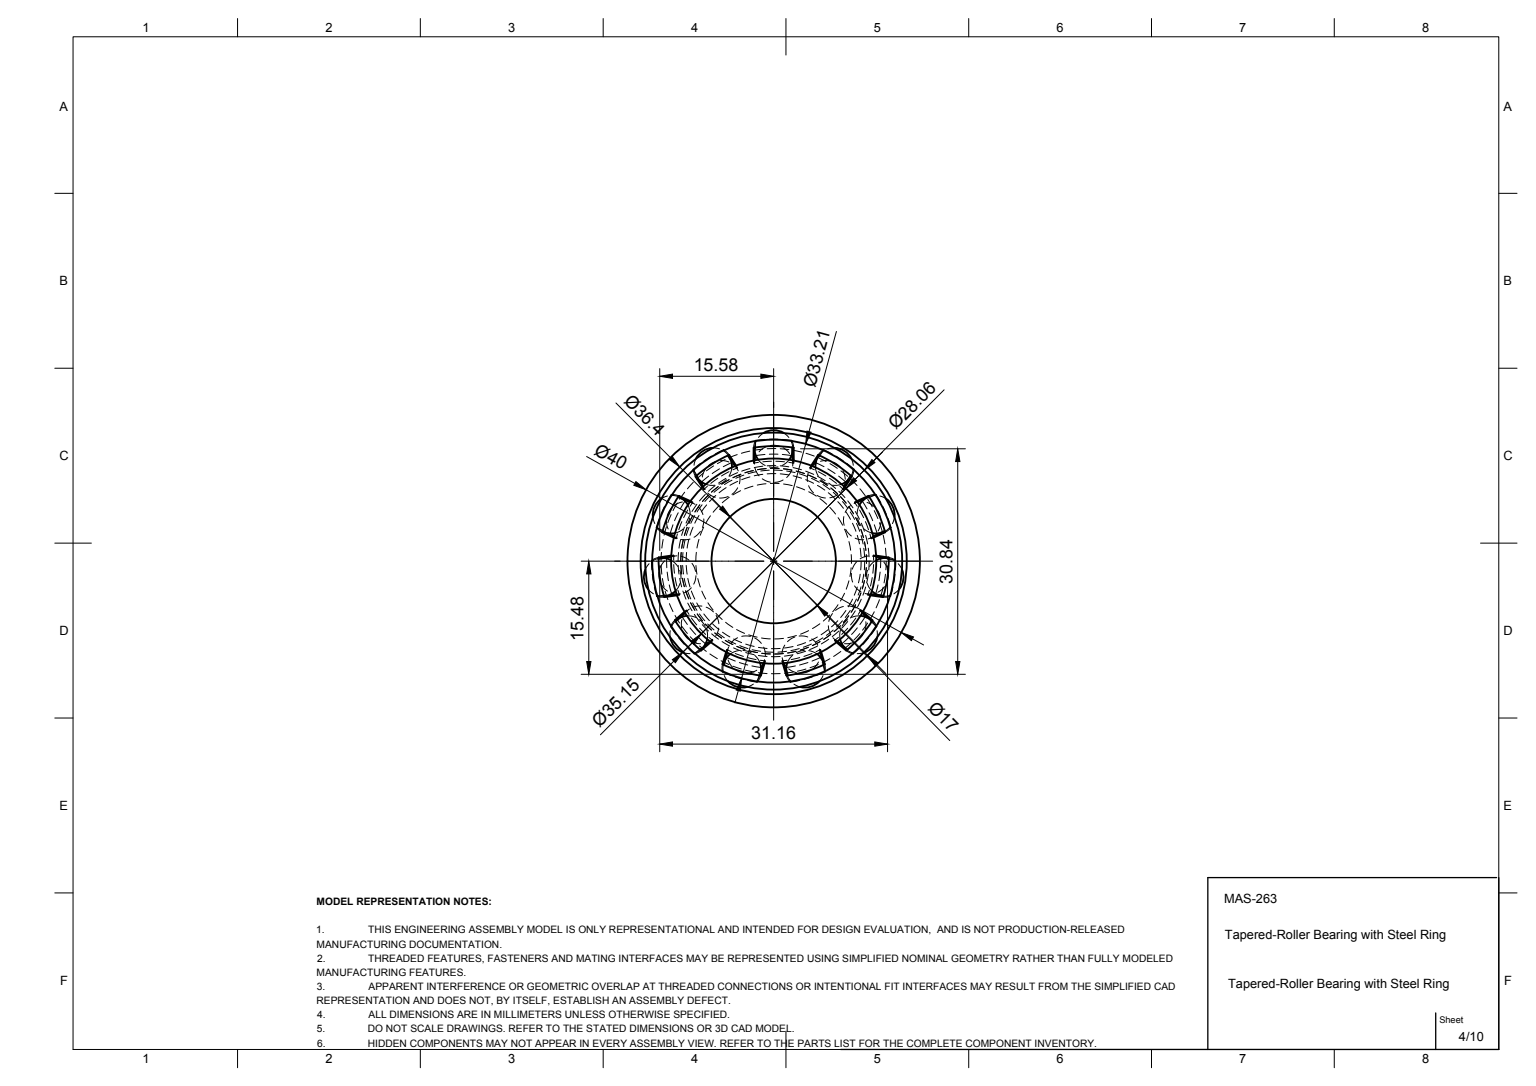
ISO-10303-21;
HEADER;
/* Generated by software containing ST-Developer
 * from STEP Tools, Inc. (www.steptools.com) 
 */

FILE_DESCRIPTION(
/* description */ (''),
/* implementation_level */ '2;1');

FILE_NAME(
/* name */ 'Tapered-Roller Bearing with Steel Ring.step',
/* time_stamp */ '2026-10-12T15:47:30-07:00',
/* author */ (''),
/* organization */ (''),
/* preprocessor_version */ 'ST-DEVELOPER v20.2',
/* originating_system */ 'Autodesk Translation Framework v15.15.0.0',
/* authorisation */ '');

FILE_SCHEMA (('AUTOMOTIVE_DESIGN { 1 0 10303 214 3 1 1 }'));
ENDSEC;

DATA;
#10=MECHANICAL_DESIGN_GEOMETRIC_PRESENTATION_REPRESENTATION('',(#103,#104,#105,#106,#107,#108,#109,#110,#111,#112,#113,#114,#115,#116),#88483);
#72=SHAPE_REPRESENTATION_RELATIONSHIP('SRR','None',#88528,#81);
#81=ADVANCED_BREP_SHAPE_REPRESENTATION('',(#138,#139,#140,#141,#142,#143,
#144,#145,#146,#147,#148,#149,#150,#151),#88482);
#103=STYLED_ITEM('',(#88574),#138);
#104=STYLED_ITEM('',(#88574),#139);
#105=STYLED_ITEM('',(#88574),#140);
#106=STYLED_ITEM('',(#88574),#141);
#107=STYLED_ITEM('',(#88574),#142);
#108=STYLED_ITEM('',(#88574),#143);
#109=STYLED_ITEM('',(#88574),#144);
#110=STYLED_ITEM('',(#88574),#145);
#111=STYLED_ITEM('',(#88574),#146);
#112=STYLED_ITEM('',(#88574),#147);
#113=STYLED_ITEM('',(#88574),#148);
#114=STYLED_ITEM('',(#88574),#149);
#115=STYLED_ITEM('',(#88574),#150);
#116=STYLED_ITEM('',(#88574),#151);
#138=MANIFOLD_SOLID_BREP('Body1',#13013);
#139=MANIFOLD_SOLID_BREP('Body2',#13014);
#140=MANIFOLD_SOLID_BREP('Body3',#13015);
#141=MANIFOLD_SOLID_BREP('Body4',#13016);
#142=MANIFOLD_SOLID_BREP('Body5',#13017);
#143=MANIFOLD_SOLID_BREP('Body6',#13018);
#144=MANIFOLD_SOLID_BREP('Body7',#13019);
#145=MANIFOLD_SOLID_BREP('Body8',#13020);
#146=MANIFOLD_SOLID_BREP('Body9',#13021);
#147=MANIFOLD_SOLID_BREP('Body10',#13022);
#148=MANIFOLD_SOLID_BREP('Body11',#13023);
#149=MANIFOLD_SOLID_BREP('Body12',#13024);
#150=MANIFOLD_SOLID_BREP('Body13',#13025);
#151=MANIFOLD_SOLID_BREP('Body14',#13026);
#185=TOROIDAL_SURFACE('',#14116,19.725,0.275);
#186=TOROIDAL_SURFACE('',#14121,19.725,0.275);
#187=TOROIDAL_SURFACE('',#14141,13.4297712445485,0.500000000000001);
#188=TOROIDAL_SURFACE('',#14288,8.775,0.275);
#189=TOROIDAL_SURFACE('',#14293,8.775,0.275);
#242=ELLIPSE('',#14151,15.0801280312954,14.5834816640173);
#243=ELLIPSE('',#14152,17.3517853554452,16.7803246128912);
#244=ELLIPSE('',#14153,17.3517853554452,16.7803246128912);
#245=ELLIPSE('',#14154,15.0801280312954,14.5834816640173);
#246=ELLIPSE('',#14155,15.0801280312954,14.5834816640173);
#247=ELLIPSE('',#14156,17.3517853554452,16.7803246128912);
#248=ELLIPSE('',#14157,17.3517853554886,16.7803246129121);
#249=ELLIPSE('',#14158,15.0801280313552,14.5834816640461);
#250=ELLIPSE('',#14159,17.351785355493,16.7803246129139);
#251=ELLIPSE('',#14160,15.0801280313139,14.5834816640261);
#252=ELLIPSE('',#14161,17.3517853552649,16.7803246128045);
#253=ELLIPSE('',#14162,15.0801280313118,14.583481664025);
#254=ELLIPSE('',#14163,17.3517853554016,16.7803246128701);
#255=ELLIPSE('',#14164,15.0801280313076,14.583481664023);
#256=ELLIPSE('',#14165,17.3517853554702,16.780324612903);
#257=ELLIPSE('',#14166,15.0801280313709,14.5834816640533);
#258=ELLIPSE('',#14167,17.3517853554861,16.7803246129107);
#259=ELLIPSE('',#14168,15.08012803127,14.583481664005);
#260=ELLIPSE('',#14169,17.3517853554707,16.7803246129033);
#261=ELLIPSE('',#14170,15.0801280312716,14.5834816640059);
#262=ELLIPSE('',#14171,17.3517853553197,16.7803246128311);
#263=ELLIPSE('',#14172,15.0801280311918,14.5834816639677);
#264=ELLIPSE('',#14173,17.3517853552856,16.7803246128146);
#265=ELLIPSE('',#14174,15.0801280313508,14.5834816640437);
#266=ELLIPSE('',#14176,18.421055935048,17.8143800174044);
#267=ELLIPSE('',#14177,16.1493986108983,15.6175370685304);
#268=ELLIPSE('',#14178,16.1493986108983,15.6175370685304);
#269=ELLIPSE('',#14179,18.421055935048,17.8143800174044);
#270=ELLIPSE('',#14180,16.1493986108983,15.6175370685304);
#271=ELLIPSE('',#14181,18.421055935048,17.8143800174044);
#272=ELLIPSE('',#14182,18.4210559352732,17.8143800175124);
#273=ELLIPSE('',#14183,16.1493986107542,15.6175370684613);
#274=ELLIPSE('',#14184,18.4210559346699,17.8143800172222);
#275=ELLIPSE('',#14185,16.1493986106406,15.6175370684066);
#276=ELLIPSE('',#14186,18.421055934899,17.8143800173331);
#277=ELLIPSE('',#14187,16.1493986106858,15.6175370684285);
#278=ELLIPSE('',#14188,18.4210559350675,17.8143800174135);
#279=ELLIPSE('',#14189,16.1493986109801,15.6175370685696);
#280=ELLIPSE('',#14190,18.4210559350065,17.8143800173844);
#281=ELLIPSE('',#14191,16.1493986108565,15.6175370685105);
#282=ELLIPSE('',#14192,18.4210559345343,17.8143800171572);
#283=ELLIPSE('',#14193,16.1493986108155,15.6175370684905);
#284=ELLIPSE('',#14194,18.4210559346994,17.8143800172367);
#285=ELLIPSE('',#14195,16.1493986107405,15.6175370684544);
#286=ELLIPSE('',#14196,18.4210559344304,17.814380017107);
#287=ELLIPSE('',#14197,16.1493986109695,15.6175370685645);
#288=ELLIPSE('',#14198,18.4210559346512,17.8143800172135);
#289=ELLIPSE('',#14199,16.1493986107542,15.6175370684612);
#337=CONICAL_SURFACE('',#14125,15.4,0.249233017184783);
#338=CONICAL_SURFACE('',#14131,12.7058184384753,1.32156330961012);
#339=CONICAL_SURFACE('',#14136,16.6071946160828,1.32156330961011);
#340=CONICAL_SURFACE('',#14146,13.3064408708579,1.32156330961011);
#341=CONICAL_SURFACE('',#14149,12.4591576910941,0.249233017184783);
#342=CONICAL_SURFACE('',#14150,13.0685506725942,0.249233017184784);
#343=CONICAL_SURFACE('',#14175,17.5762965073726,0.249233017184784);
#344=CONICAL_SURFACE('',#14297,10.6410293263727,1.32156330961011);
#345=CONICAL_SURFACE('',#14301,12.6998790237181,0.249233017184785);
#346=CONICAL_SURFACE('',#14304,14.0317131491268,1.32156330961011);
#416=FACE_BOUND('',#2102,.T.);
#417=FACE_BOUND('',#2104,.T.);
#418=FACE_BOUND('',#2111,.T.);
#419=FACE_BOUND('',#2112,.T.);
#420=FACE_BOUND('',#2113,.T.);
#421=FACE_BOUND('',#2114,.T.);
#422=FACE_BOUND('',#2115,.T.);
#423=FACE_BOUND('',#2116,.T.);
#424=FACE_BOUND('',#2117,.T.);
#425=FACE_BOUND('',#2118,.T.);
#426=FACE_BOUND('',#2119,.T.);
#427=FACE_BOUND('',#2120,.T.);
#428=FACE_BOUND('',#2122,.T.);
#429=FACE_BOUND('',#2123,.T.);
#430=FACE_BOUND('',#2124,.T.);
#431=FACE_BOUND('',#2125,.T.);
#432=FACE_BOUND('',#2126,.T.);
#433=FACE_BOUND('',#2127,.T.);
#434=FACE_BOUND('',#2128,.T.);
#435=FACE_BOUND('',#2129,.T.);
#436=FACE_BOUND('',#2130,.T.);
#437=FACE_BOUND('',#2131,.T.);
#438=FACE_BOUND('',#2185,.T.);
#439=FACE_BOUND('',#2187,.T.);
#562=PLANE('',#14129);
#563=PLANE('',#14130);
#564=PLANE('',#14206);
#565=PLANE('',#14207);
#566=PLANE('',#14214);
#567=PLANE('',#14215);
#568=PLANE('',#14222);
#569=PLANE('',#14223);
#570=PLANE('',#14230);
#571=PLANE('',#14231);
#572=PLANE('',#14238);
#573=PLANE('',#14239);
#574=PLANE('',#14246);
#575=PLANE('',#14247);
#576=PLANE('',#14254);
#577=PLANE('',#14255);
#578=PLANE('',#14262);
#579=PLANE('',#14263);
#580=PLANE('',#14270);
#581=PLANE('',#14271);
#582=PLANE('',#14278);
#583=PLANE('',#14279);
#584=PLANE('',#14286);
#585=PLANE('',#14287);
#586=PLANE('',#14311);
#587=PLANE('',#14312);
#588=PLANE('',#14316);
#589=PLANE('',#14317);
#590=PLANE('',#14321);
#591=PLANE('',#14322);
#592=PLANE('',#14326);
#593=PLANE('',#14327);
#594=PLANE('',#14331);
#595=PLANE('',#14332);
#596=PLANE('',#14336);
#597=PLANE('',#14337);
#598=PLANE('',#14341);
#599=PLANE('',#14342);
#600=PLANE('',#14346);
#601=PLANE('',#14347);
#602=PLANE('',#14351);
#603=PLANE('',#14352);
#604=PLANE('',#14356);
#605=PLANE('',#14357);
#606=PLANE('',#14361);
#607=PLANE('',#14362);
#608=PLANE('',#14366);
#609=PLANE('',#14367);
#1362=FACE_OUTER_BOUND('',#2097,.T.);
#1363=FACE_OUTER_BOUND('',#2098,.T.);
#1364=FACE_OUTER_BOUND('',#2099,.T.);
#1365=FACE_OUTER_BOUND('',#2100,.T.);
#1366=FACE_OUTER_BOUND('',#2101,.T.);
#1367=FACE_OUTER_BOUND('',#2103,.T.);
#1368=FACE_OUTER_BOUND('',#2105,.T.);
#1369=FACE_OUTER_BOUND('',#2106,.T.);
#1370=FACE_OUTER_BOUND('',#2107,.T.);
#1371=FACE_OUTER_BOUND('',#2108,.T.);
#1372=FACE_OUTER_BOUND('',#2109,.T.);
#1373=FACE_OUTER_BOUND('',#2110,.T.);
#1374=FACE_OUTER_BOUND('',#2121,.T.);
#1375=FACE_OUTER_BOUND('',#2132,.T.);
#1376=FACE_OUTER_BOUND('',#2133,.T.);
#1377=FACE_OUTER_BOUND('',#2134,.T.);
#1378=FACE_OUTER_BOUND('',#2135,.T.);
#1379=FACE_OUTER_BOUND('',#2136,.T.);
#1380=FACE_OUTER_BOUND('',#2137,.T.);
#1381=FACE_OUTER_BOUND('',#2138,.T.);
#1382=FACE_OUTER_BOUND('',#2139,.T.);
#1383=FACE_OUTER_BOUND('',#2140,.T.);
#1384=FACE_OUTER_BOUND('',#2141,.T.);
#1385=FACE_OUTER_BOUND('',#2142,.T.);
#1386=FACE_OUTER_BOUND('',#2143,.T.);
#1387=FACE_OUTER_BOUND('',#2144,.T.);
#1388=FACE_OUTER_BOUND('',#2145,.T.);
#1389=FACE_OUTER_BOUND('',#2146,.T.);
#1390=FACE_OUTER_BOUND('',#2147,.T.);
#1391=FACE_OUTER_BOUND('',#2148,.T.);
#1392=FACE_OUTER_BOUND('',#2149,.T.);
#1393=FACE_OUTER_BOUND('',#2150,.T.);
#1394=FACE_OUTER_BOUND('',#2151,.T.);
#1395=FACE_OUTER_BOUND('',#2152,.T.);
#1396=FACE_OUTER_BOUND('',#2153,.T.);
#1397=FACE_OUTER_BOUND('',#2154,.T.);
#1398=FACE_OUTER_BOUND('',#2155,.T.);
#1399=FACE_OUTER_BOUND('',#2156,.T.);
#1400=FACE_OUTER_BOUND('',#2157,.T.);
#1401=FACE_OUTER_BOUND('',#2158,.T.);
#1402=FACE_OUTER_BOUND('',#2159,.T.);
#1403=FACE_OUTER_BOUND('',#2160,.T.);
#1404=FACE_OUTER_BOUND('',#2161,.T.);
#1405=FACE_OUTER_BOUND('',#2162,.T.);
#1406=FACE_OUTER_BOUND('',#2163,.T.);
#1407=FACE_OUTER_BOUND('',#2164,.T.);
#1408=FACE_OUTER_BOUND('',#2165,.T.);
#1409=FACE_OUTER_BOUND('',#2166,.T.);
#1410=FACE_OUTER_BOUND('',#2167,.T.);
#1411=FACE_OUTER_BOUND('',#2168,.T.);
#1412=FACE_OUTER_BOUND('',#2169,.T.);
#1413=FACE_OUTER_BOUND('',#2170,.T.);
#1414=FACE_OUTER_BOUND('',#2171,.T.);
#1415=FACE_OUTER_BOUND('',#2172,.T.);
#1416=FACE_OUTER_BOUND('',#2173,.T.);
#1417=FACE_OUTER_BOUND('',#2174,.T.);
#1418=FACE_OUTER_BOUND('',#2175,.T.);
#1419=FACE_OUTER_BOUND('',#2176,.T.);
#1420=FACE_OUTER_BOUND('',#2177,.T.);
#1421=FACE_OUTER_BOUND('',#2178,.T.);
#1422=FACE_OUTER_BOUND('',#2179,.T.);
#1423=FACE_OUTER_BOUND('',#2180,.T.);
#1424=FACE_OUTER_BOUND('',#2181,.T.);
#1425=FACE_OUTER_BOUND('',#2182,.T.);
#1426=FACE_OUTER_BOUND('',#2183,.T.);
#1427=FACE_OUTER_BOUND('',#2184,.T.);
#1428=FACE_OUTER_BOUND('',#2186,.T.);
#1429=FACE_OUTER_BOUND('',#2188,.T.);
#1430=FACE_OUTER_BOUND('',#2189,.T.);
#1431=FACE_OUTER_BOUND('',#2190,.T.);
#1432=FACE_OUTER_BOUND('',#2191,.T.);
#1433=FACE_OUTER_BOUND('',#2192,.T.);
#1434=FACE_OUTER_BOUND('',#2193,.T.);
#1435=FACE_OUTER_BOUND('',#2194,.T.);
#1436=FACE_OUTER_BOUND('',#2195,.T.);
#1437=FACE_OUTER_BOUND('',#2196,.T.);
#1438=FACE_OUTER_BOUND('',#2197,.T.);
#1439=FACE_OUTER_BOUND('',#2198,.T.);
#1440=FACE_OUTER_BOUND('',#2199,.T.);
#1441=FACE_OUTER_BOUND('',#2200,.T.);
#1442=FACE_OUTER_BOUND('',#2201,.T.);
#1443=FACE_OUTER_BOUND('',#2202,.T.);
#1444=FACE_OUTER_BOUND('',#2203,.T.);
#1445=FACE_OUTER_BOUND('',#2204,.T.);
#1446=FACE_OUTER_BOUND('',#2205,.T.);
#1447=FACE_OUTER_BOUND('',#2206,.T.);
#1448=FACE_OUTER_BOUND('',#2207,.T.);
#1449=FACE_OUTER_BOUND('',#2208,.T.);
#1450=FACE_OUTER_BOUND('',#2209,.T.);
#1451=FACE_OUTER_BOUND('',#2210,.T.);
#1452=FACE_OUTER_BOUND('',#2211,.T.);
#1453=FACE_OUTER_BOUND('',#2212,.T.);
#1454=FACE_OUTER_BOUND('',#2213,.T.);
#1455=FACE_OUTER_BOUND('',#2214,.T.);
#1456=FACE_OUTER_BOUND('',#2215,.T.);
#1457=FACE_OUTER_BOUND('',#2216,.T.);
#1458=FACE_OUTER_BOUND('',#2217,.T.);
#1459=FACE_OUTER_BOUND('',#2218,.T.);
#1460=FACE_OUTER_BOUND('',#2219,.T.);
#1461=FACE_OUTER_BOUND('',#2220,.T.);
#2097=EDGE_LOOP('',(#11674,#11675,#11676,#11677,#11678));
#2098=EDGE_LOOP('',(#11679,#11680,#11681,#11682));
#2099=EDGE_LOOP('',(#11683,#11684,#11685,#11686));
#2100=EDGE_LOOP('',(#11687,#11688,#11689,#11690,#11691));
#2101=EDGE_LOOP('',(#11692));
#2102=EDGE_LOOP('',(#11693));
#2103=EDGE_LOOP('',(#11694));
#2104=EDGE_LOOP('',(#11695));
#2105=EDGE_LOOP('',(#11696,#11697,#11698,#11699,#11700,#11701));
#2106=EDGE_LOOP('',(#11702,#11703,#11704,#11705,#11706,#11707));
#2107=EDGE_LOOP('',(#11708,#11709,#11710,#11711,#11712));
#2108=EDGE_LOOP('',(#11713,#11714,#11715,#11716,#11717));
#2109=EDGE_LOOP('',(#11718,#11719,#11720,#11721,#11722,#11723));
#2110=EDGE_LOOP('',(#11724,#11725,#11726,#11727,#11728,#11729,#11730,#11731,
#11732,#11733,#11734,#11735,#11736,#11737));
#2111=EDGE_LOOP('',(#11738,#11739,#11740,#11741));
#2112=EDGE_LOOP('',(#11742,#11743,#11744,#11745));
#2113=EDGE_LOOP('',(#11746,#11747,#11748,#11749));
#2114=EDGE_LOOP('',(#11750,#11751,#11752,#11753));
#2115=EDGE_LOOP('',(#11754,#11755,#11756,#11757));
#2116=EDGE_LOOP('',(#11758,#11759,#11760,#11761));
#2117=EDGE_LOOP('',(#11762,#11763,#11764,#11765));
#2118=EDGE_LOOP('',(#11766,#11767,#11768,#11769));
#2119=EDGE_LOOP('',(#11770,#11771,#11772,#11773));
#2120=EDGE_LOOP('',(#11774,#11775,#11776,#11777));
#2121=EDGE_LOOP('',(#11778,#11779,#11780,#11781,#11782,#11783,#11784,#11785,
#11786,#11787,#11788,#11789,#11790,#11791));
#2122=EDGE_LOOP('',(#11792,#11793,#11794,#11795));
#2123=EDGE_LOOP('',(#11796,#11797,#11798,#11799));
#2124=EDGE_LOOP('',(#11800,#11801,#11802,#11803));
#2125=EDGE_LOOP('',(#11804,#11805,#11806,#11807));
#2126=EDGE_LOOP('',(#11808,#11809,#11810,#11811));
#2127=EDGE_LOOP('',(#11812,#11813,#11814,#11815));
#2128=EDGE_LOOP('',(#11816,#11817,#11818,#11819));
#2129=EDGE_LOOP('',(#11820,#11821,#11822,#11823));
#2130=EDGE_LOOP('',(#11824,#11825,#11826,#11827));
#2131=EDGE_LOOP('',(#11828,#11829,#11830,#11831));
#2132=EDGE_LOOP('',(#11832,#11833,#11834,#11835));
#2133=EDGE_LOOP('',(#11836,#11837,#11838,#11839));
#2134=EDGE_LOOP('',(#11840,#11841,#11842,#11843));
#2135=EDGE_LOOP('',(#11844,#11845,#11846,#11847));
#2136=EDGE_LOOP('',(#11848,#11849,#11850,#11851));
#2137=EDGE_LOOP('',(#11852,#11853,#11854,#11855));
#2138=EDGE_LOOP('',(#11856,#11857,#11858,#11859));
#2139=EDGE_LOOP('',(#11860,#11861,#11862,#11863));
#2140=EDGE_LOOP('',(#11864,#11865,#11866,#11867));
#2141=EDGE_LOOP('',(#11868,#11869,#11870,#11871));
#2142=EDGE_LOOP('',(#11872,#11873,#11874,#11875));
#2143=EDGE_LOOP('',(#11876,#11877,#11878,#11879));
#2144=EDGE_LOOP('',(#11880,#11881,#11882,#11883));
#2145=EDGE_LOOP('',(#11884,#11885,#11886,#11887));
#2146=EDGE_LOOP('',(#11888,#11889,#11890,#11891));
#2147=EDGE_LOOP('',(#11892,#11893,#11894,#11895));
#2148=EDGE_LOOP('',(#11896,#11897,#11898,#11899));
#2149=EDGE_LOOP('',(#11900,#11901,#11902,#11903));
#2150=EDGE_LOOP('',(#11904,#11905,#11906,#11907));
#2151=EDGE_LOOP('',(#11908,#11909,#11910,#11911));
#2152=EDGE_LOOP('',(#11912,#11913,#11914,#11915));
#2153=EDGE_LOOP('',(#11916,#11917,#11918,#11919));
#2154=EDGE_LOOP('',(#11920,#11921,#11922,#11923));
#2155=EDGE_LOOP('',(#11924,#11925,#11926,#11927));
#2156=EDGE_LOOP('',(#11928,#11929,#11930,#11931));
#2157=EDGE_LOOP('',(#11932,#11933,#11934,#11935));
#2158=EDGE_LOOP('',(#11936,#11937,#11938,#11939));
#2159=EDGE_LOOP('',(#11940,#11941,#11942,#11943));
#2160=EDGE_LOOP('',(#11944,#11945,#11946,#11947));
#2161=EDGE_LOOP('',(#11948,#11949,#11950,#11951));
#2162=EDGE_LOOP('',(#11952,#11953,#11954,#11955));
#2163=EDGE_LOOP('',(#11956,#11957,#11958,#11959));
#2164=EDGE_LOOP('',(#11960,#11961,#11962,#11963));
#2165=EDGE_LOOP('',(#11964,#11965,#11966,#11967));
#2166=EDGE_LOOP('',(#11968,#11969,#11970,#11971));
#2167=EDGE_LOOP('',(#11972,#11973,#11974,#11975));
#2168=EDGE_LOOP('',(#11976,#11977,#11978,#11979));
#2169=EDGE_LOOP('',(#11980,#11981,#11982,#11983));
#2170=EDGE_LOOP('',(#11984,#11985,#11986,#11987,#11988,#11989));
#2171=EDGE_LOOP('',(#11990,#11991,#11992,#11993,#11994,#11995));
#2172=EDGE_LOOP('',(#11996,#11997,#11998,#11999));
#2173=EDGE_LOOP('',(#12000,#12001,#12002,#12003));
#2174=EDGE_LOOP('',(#12004,#12005,#12006,#12007));
#2175=EDGE_LOOP('',(#12008,#12009,#12010,#12011));
#2176=EDGE_LOOP('',(#12012,#12013,#12014,#12015,#12016));
#2177=EDGE_LOOP('',(#12017,#12018,#12019,#12020));
#2178=EDGE_LOOP('',(#12021,#12022,#12023,#12024,#12025));
#2179=EDGE_LOOP('',(#12026,#12027,#12028,#12029,#12030,#12031));
#2180=EDGE_LOOP('',(#12032,#12033,#12034,#12035,#12036));
#2181=EDGE_LOOP('',(#12037,#12038,#12039,#12040));
#2182=EDGE_LOOP('',(#12041,#12042,#12043,#12044,#12045));
#2183=EDGE_LOOP('',(#12046,#12047,#12048,#12049));
#2184=EDGE_LOOP('',(#12050));
#2185=EDGE_LOOP('',(#12051));
#2186=EDGE_LOOP('',(#12052));
#2187=EDGE_LOOP('',(#12053));
#2188=EDGE_LOOP('',(#12054,#12055,#12056,#12057));
#2189=EDGE_LOOP('',(#12058));
#2190=EDGE_LOOP('',(#12059));
#2191=EDGE_LOOP('',(#12060,#12061,#12062,#12063));
#2192=EDGE_LOOP('',(#12064));
#2193=EDGE_LOOP('',(#12065));
#2194=EDGE_LOOP('',(#12066,#12067,#12068,#12069));
#2195=EDGE_LOOP('',(#12070));
#2196=EDGE_LOOP('',(#12071));
#2197=EDGE_LOOP('',(#12072,#12073,#12074,#12075));
#2198=EDGE_LOOP('',(#12076));
#2199=EDGE_LOOP('',(#12077));
#2200=EDGE_LOOP('',(#12078,#12079,#12080,#12081));
#2201=EDGE_LOOP('',(#12082));
#2202=EDGE_LOOP('',(#12083));
#2203=EDGE_LOOP('',(#12084,#12085,#12086,#12087));
#2204=EDGE_LOOP('',(#12088));
#2205=EDGE_LOOP('',(#12089));
#2206=EDGE_LOOP('',(#12090,#12091,#12092,#12093));
#2207=EDGE_LOOP('',(#12094));
#2208=EDGE_LOOP('',(#12095));
#2209=EDGE_LOOP('',(#12096,#12097,#12098,#12099));
#2210=EDGE_LOOP('',(#12100));
#2211=EDGE_LOOP('',(#12101));
#2212=EDGE_LOOP('',(#12102,#12103,#12104,#12105));
#2213=EDGE_LOOP('',(#12106));
#2214=EDGE_LOOP('',(#12107));
#2215=EDGE_LOOP('',(#12108,#12109,#12110,#12111));
#2216=EDGE_LOOP('',(#12112));
#2217=EDGE_LOOP('',(#12113));
#2218=EDGE_LOOP('',(#12114,#12115,#12116,#12117));
#2219=EDGE_LOOP('',(#12118));
#2220=EDGE_LOOP('',(#12119));
#2768=CIRCLE('',#14117,20.);
#2769=CIRCLE('',#14118,20.);
#2770=CIRCLE('',#14119,0.275);
#2771=CIRCLE('',#14120,19.725);
#2772=CIRCLE('',#14122,20.);
#2773=CIRCLE('',#14123,0.275);
#2774=CIRCLE('',#14124,19.725);
#2775=CIRCLE('',#14126,15.4);
#2776=CIRCLE('',#14127,18.1997760045464);
#2777=CIRCLE('',#14132,13.0685506725942);
#2778=CIRCLE('',#14133,13.0685506725942);
#2779=CIRCLE('',#14134,12.7058184384753);
#2780=CIRCLE('',#14135,12.7058184384753);
#2781=CIRCLE('',#14137,17.5762965073726);
#2782=CIRCLE('',#14138,17.5762965073726);
#2783=CIRCLE('',#14139,16.6071946160828);
#2784=CIRCLE('',#14140,16.6071946160828);
#2785=CIRCLE('',#14142,13.3064408708579);
#2786=CIRCLE('',#14143,0.500000000000001);
#2787=CIRCLE('',#14144,13.9143221901933);
#2788=CIRCLE('',#14145,13.9143221901933);
#2789=CIRCLE('',#14147,12.4591576910941);
#2790=CIRCLE('',#14148,12.4591576910941);
#2791=CIRCLE('',#14201,2.74859462638384);
#2792=CIRCLE('',#14202,2.74859462638384);
#2793=CIRCLE('',#14204,2.74859462638384);
#2794=CIRCLE('',#14205,2.74859462638384);
#2795=CIRCLE('',#14209,2.74859462638384);
#2796=CIRCLE('',#14210,2.74859462638384);
#2797=CIRCLE('',#14212,2.74859462638384);
#2798=CIRCLE('',#14213,2.74859462638384);
#2799=CIRCLE('',#14217,2.74859462638385);
#2800=CIRCLE('',#14218,2.74859462638384);
#2801=CIRCLE('',#14220,2.74859462638384);
#2802=CIRCLE('',#14221,2.74859462638385);
#2803=CIRCLE('',#14225,2.74859462638384);
#2804=CIRCLE('',#14226,2.74859462638384);
#2805=CIRCLE('',#14228,2.74859462638384);
#2806=CIRCLE('',#14229,2.74859462638384);
#2807=CIRCLE('',#14233,2.74859462638384);
#2808=CIRCLE('',#14234,2.74859462638384);
#2809=CIRCLE('',#14236,2.74859462638384);
#2810=CIRCLE('',#14237,2.74859462638384);
#2811=CIRCLE('',#14241,2.74859462638384);
#2812=CIRCLE('',#14242,2.74859462638384);
#2813=CIRCLE('',#14244,2.74859462638384);
#2814=CIRCLE('',#14245,2.74859462638384);
#2815=CIRCLE('',#14249,2.74859462638384);
#2816=CIRCLE('',#14250,2.74859462638384);
#2817=CIRCLE('',#14252,2.74859462638384);
#2818=CIRCLE('',#14253,2.74859462638384);
#2819=CIRCLE('',#14257,2.74859462638384);
#2820=CIRCLE('',#14258,2.74859462638384);
#2821=CIRCLE('',#14260,2.74859462638384);
#2822=CIRCLE('',#14261,2.74859462638384);
#2823=CIRCLE('',#14265,2.74859462638384);
#2824=CIRCLE('',#14266,2.74859462638384);
#2825=CIRCLE('',#14268,2.74859462638384);
#2826=CIRCLE('',#14269,2.74859462638384);
#2827=CIRCLE('',#14273,2.74859462638384);
#2828=CIRCLE('',#14274,2.74859462638384);
#2829=CIRCLE('',#14276,2.74859462638384);
#2830=CIRCLE('',#14277,2.74859462638384);
#2831=CIRCLE('',#14281,2.74859462638384);
#2832=CIRCLE('',#14282,2.74859462638384);
#2833=CIRCLE('',#14284,2.74859462638384);
#2834=CIRCLE('',#14285,2.74859462638384);
#2835=CIRCLE('',#14289,8.775);
#2836=CIRCLE('',#14290,0.275);
#2837=CIRCLE('',#14291,8.5);
#2838=CIRCLE('',#14292,8.5);
#2839=CIRCLE('',#14294,8.775);
#2840=CIRCLE('',#14295,0.275);
#2841=CIRCLE('',#14296,8.5);
#2842=CIRCLE('',#14298,11.9728634517814);
#2843=CIRCLE('',#14299,10.6410293263727);
#2844=CIRCLE('',#14300,10.6410293263727);
#2845=CIRCLE('',#14302,12.6998790237181);
#2846=CIRCLE('',#14303,12.6998790237181);
#2847=CIRCLE('',#14305,14.0317131491268);
#2848=CIRCLE('',#14307,14.0317131491268);
#2849=CIRCLE('',#14310,11.9728634517814);
#2850=CIRCLE('',#14314,2.62159462638384);
#2851=CIRCLE('',#14315,2.62159462638384);
#2852=CIRCLE('',#14319,2.62159462638384);
#2853=CIRCLE('',#14320,2.62159462638384);
#2854=CIRCLE('',#14324,2.62159462638384);
#2855=CIRCLE('',#14325,2.62159462638384);
#2856=CIRCLE('',#14329,2.62159462638384);
#2857=CIRCLE('',#14330,2.62159462638384);
#2858=CIRCLE('',#14334,2.62159462638384);
#2859=CIRCLE('',#14335,2.62159462638384);
#2860=CIRCLE('',#14339,2.62159462638384);
#2861=CIRCLE('',#14340,2.62159462638384);
#2862=CIRCLE('',#14344,2.62159462638384);
#2863=CIRCLE('',#14345,2.62159462638384);
#2864=CIRCLE('',#14349,2.62159462638384);
#2865=CIRCLE('',#14350,2.62159462638384);
#2866=CIRCLE('',#14354,2.62159462638384);
#2867=CIRCLE('',#14355,2.62159462638384);
#2868=CIRCLE('',#14359,2.62159462638384);
#2869=CIRCLE('',#14360,2.62159462638384);
#2870=CIRCLE('',#14364,2.62159462638384);
#2871=CIRCLE('',#14365,2.62159462638384);
#3631=B_SPLINE_CURVE_WITH_KNOTS('',3,(#87783,#87784,#87785,#87786,#87787,
#87788,#87789),.UNSPECIFIED.,.F.,.F.,(4,3,4),(0.000674089299982974,0.00549718988211594,
0.00902105606223609),.UNSPECIFIED.);
#3632=B_SPLINE_CURVE_WITH_KNOTS('',3,(#87796,#87797,#87798,#87799,#87800,
#87801,#87802),.UNSPECIFIED.,.F.,.F.,(4,3,4),(0.000736267499631611,0.00549718958832386,
0.00908323445073435),.UNSPECIFIED.);
#3633=B_SPLINE_CURVE_WITH_KNOTS('',3,(#87808,#87809,#87810,#87811,#87812,
#87813,#87814),.UNSPECIFIED.,.F.,.F.,(4,3,4),(0.000674089299982975,0.00549718988211594,
0.00902105608511028),.UNSPECIFIED.);
#3634=B_SPLINE_CURVE_WITH_KNOTS('',3,(#87817,#87818,#87819,#87820,#87821,
#87822,#87823),.UNSPECIFIED.,.F.,.F.,(4,3,4),(0.000300808474506944,0.00549718960300923,
0.0086477753818904),.UNSPECIFIED.);
#3635=B_SPLINE_CURVE_WITH_KNOTS('',3,(#87828,#87829,#87830,#87831,#87832,
#87833,#87834),.UNSPECIFIED.,.F.,.F.,(4,3,4),(0.00073626749963161,0.00549718958832386,
0.00908323445073435),.UNSPECIFIED.);
#3636=B_SPLINE_CURVE_WITH_KNOTS('',3,(#87837,#87838,#87839,#87840,#87841,
#87842,#87843),.UNSPECIFIED.,.F.,.F.,(4,3,4),(0.000674089299982974,0.00549718988211594,
0.00902105608511028),.UNSPECIFIED.);
#3637=B_SPLINE_CURVE_WITH_KNOTS('',3,(#87848,#87849,#87850,#87851,#87852,
#87853,#87854),.UNSPECIFIED.,.F.,.F.,(4,3,4),(0.000736267499631611,0.00549718958832386,
0.00908323445073436),.UNSPECIFIED.);
#3638=B_SPLINE_CURVE_WITH_KNOTS('',3,(#87857,#87858,#87859,#87860,#87861,
#87862,#87863),.UNSPECIFIED.,.F.,.F.,(4,3,4),(0.000674089299982974,0.00549718988211594,
0.00902105608511028),.UNSPECIFIED.);
#3639=B_SPLINE_CURVE_WITH_KNOTS('',3,(#87868,#87869,#87870,#87871,#87872,
#87873,#87874),.UNSPECIFIED.,.F.,.F.,(4,3,4),(0.00073626749963161,0.00549718958832386,
0.00908323445073435),.UNSPECIFIED.);
#3640=B_SPLINE_CURVE_WITH_KNOTS('',3,(#87877,#87878,#87879,#87880,#87881,
#87882,#87883),.UNSPECIFIED.,.F.,.F.,(4,3,4),(0.000674089299982977,0.00549718988211594,
0.00902105608511028),.UNSPECIFIED.);
#3641=B_SPLINE_CURVE_WITH_KNOTS('',3,(#87888,#87889,#87890,#87891,#87892,
#87893,#87894),.UNSPECIFIED.,.F.,.F.,(4,3,4),(0.000736267499631609,0.00549718958832386,
0.00908323445073436),.UNSPECIFIED.);
#3642=B_SPLINE_CURVE_WITH_KNOTS('',3,(#87897,#87898,#87899,#87900,#87901,
#87902,#87903),.UNSPECIFIED.,.F.,.F.,(4,3,4),(0.000674089299982975,0.00549718988211594,
0.00902105608511028),.UNSPECIFIED.);
#3643=B_SPLINE_CURVE_WITH_KNOTS('',3,(#87908,#87909,#87910,#87911,#87912,
#87913,#87914),.UNSPECIFIED.,.F.,.F.,(4,3,4),(0.00073626749963161,0.00549718958832386,
0.00908323445073436),.UNSPECIFIED.);
#3644=B_SPLINE_CURVE_WITH_KNOTS('',3,(#87917,#87918,#87919,#87920,#87921,
#87922,#87923),.UNSPECIFIED.,.F.,.F.,(4,3,4),(0.000674089299982974,0.00549718988211594,
0.00902105608511028),.UNSPECIFIED.);
#3645=B_SPLINE_CURVE_WITH_KNOTS('',3,(#87928,#87929,#87930,#87931,#87932,
#87933,#87934),.UNSPECIFIED.,.F.,.F.,(4,3,4),(0.00073626749963161,0.00549718958832386,
0.00908323445073435),.UNSPECIFIED.);
#3646=B_SPLINE_CURVE_WITH_KNOTS('',3,(#87937,#87938,#87939,#87940,#87941,
#87942,#87943),.UNSPECIFIED.,.F.,.F.,(4,3,4),(0.000674089299982975,0.00549718988211594,
0.00902105608511028),.UNSPECIFIED.);
#3647=B_SPLINE_CURVE_WITH_KNOTS('',3,(#87948,#87949,#87950,#87951,#87952,
#87953,#87954),.UNSPECIFIED.,.F.,.F.,(4,3,4),(0.00073626749963161,0.00549718958832386,
0.00908323445073435),.UNSPECIFIED.);
#3648=B_SPLINE_CURVE_WITH_KNOTS('',3,(#87957,#87958,#87959,#87960,#87961,
#87962,#87963),.UNSPECIFIED.,.F.,.F.,(4,3,4),(0.000674089299982974,0.00549718988211594,
0.00902105608511028),.UNSPECIFIED.);
#3649=B_SPLINE_CURVE_WITH_KNOTS('',3,(#87968,#87969,#87970,#87971,#87972,
#87973,#87974),.UNSPECIFIED.,.F.,.F.,(4,3,4),(0.000736267499631611,0.00549718958832386,
0.00908323445073436),.UNSPECIFIED.);
#3650=B_SPLINE_CURVE_WITH_KNOTS('',3,(#87977,#87978,#87979,#87980,#87981,
#87982,#87983),.UNSPECIFIED.,.F.,.F.,(4,3,4),(0.000674089299982975,0.00549718988211594,
0.00902105608511028),.UNSPECIFIED.);
#3651=B_SPLINE_CURVE_WITH_KNOTS('',3,(#87988,#87989,#87990,#87991,#87992,
#87993,#87994),.UNSPECIFIED.,.F.,.F.,(4,3,4),(0.000736267499631609,0.00549718958832386,
0.00908323445073436),.UNSPECIFIED.);
#3652=B_SPLINE_CURVE_WITH_KNOTS('',3,(#87997,#87998,#87999,#88000,#88001,
#88002,#88003),.UNSPECIFIED.,.F.,.F.,(4,3,4),(0.000674089299982975,0.00549718988211594,
0.00902105608511028),.UNSPECIFIED.);
#3653=B_SPLINE_CURVE_WITH_KNOTS('',3,(#88010,#88011,#88012,#88013,#88014,
#88015,#88016),.UNSPECIFIED.,.F.,.F.,(4,3,4),(0.0010048444099522,0.00549718948033446,
0.00935178896934134),.UNSPECIFIED.);
#3654=B_SPLINE_CURVE_WITH_KNOTS('',3,(#88023,#88024,#88025,#88026,#88027,
#88028,#88029),.UNSPECIFIED.,.F.,.F.,(4,3,4),(0.000402895054555106,0.00549718967396158,
0.00874983950741581),.UNSPECIFIED.);
#3655=B_SPLINE_CURVE_WITH_KNOTS('',3,(#88035,#88036,#88037,#88038,#88039,
#88040,#88041),.UNSPECIFIED.,.F.,.F.,(4,3,4),(0.000402895054555106,0.00549718967396158,
0.00874983950741581),.UNSPECIFIED.);
#3656=B_SPLINE_CURVE_WITH_KNOTS('',3,(#88044,#88045,#88046,#88047,#88048,
#88049,#88050),.UNSPECIFIED.,.F.,.F.,(4,3,4),(0.0010048444099522,0.00549718948033446,
0.00935178896934134),.UNSPECIFIED.);
#3657=B_SPLINE_CURVE_WITH_KNOTS('',3,(#88055,#88056,#88057,#88058,#88059,
#88060,#88061),.UNSPECIFIED.,.F.,.F.,(4,3,4),(0.000514450719951176,0.00549718949135943,
0.00886139524895251),.UNSPECIFIED.);
#3658=B_SPLINE_CURVE_WITH_KNOTS('',3,(#88064,#88065,#88066,#88067,#88068,
#88069,#88070),.UNSPECIFIED.,.F.,.F.,(4,3,4),(0.000402895054555106,0.00549718967396158,
0.00874983950741581),.UNSPECIFIED.);
#3659=B_SPLINE_CURVE_WITH_KNOTS('',3,(#88075,#88076,#88077,#88078,#88079,
#88080,#88081),.UNSPECIFIED.,.F.,.F.,(4,3,4),(0.000595284717236738,0.00549718948949992,
0.00894222925114684),.UNSPECIFIED.);
#3660=B_SPLINE_CURVE_WITH_KNOTS('',3,(#88084,#88085,#88086,#88087,#88088,
#88089,#88090),.UNSPECIFIED.,.F.,.F.,(4,3,4),(0.000402895054555105,0.00549718967396158,
0.00874983950741581),.UNSPECIFIED.);
#3661=B_SPLINE_CURVE_WITH_KNOTS('',3,(#88095,#88096,#88097,#88098,#88099,
#88100,#88101),.UNSPECIFIED.,.F.,.F.,(4,3,4),(0.0010048444099522,0.00549718948033446,
0.00935178896934135),.UNSPECIFIED.);
#3662=B_SPLINE_CURVE_WITH_KNOTS('',3,(#88104,#88105,#88106,#88107,#88108,
#88109,#88110),.UNSPECIFIED.,.F.,.F.,(4,3,4),(0.000402895054555106,0.00549718967396158,
0.00874983949247052),.UNSPECIFIED.);
#3663=B_SPLINE_CURVE_WITH_KNOTS('',3,(#88115,#88116,#88117,#88118,#88119,
#88120,#88121),.UNSPECIFIED.,.F.,.F.,(4,3,4),(0.0010048444099522,0.00549718948033446,
0.00935178896934134),.UNSPECIFIED.);
#3664=B_SPLINE_CURVE_WITH_KNOTS('',3,(#88124,#88125,#88126,#88127,#88128,
#88129,#88130),.UNSPECIFIED.,.F.,.F.,(4,3,4),(0.000402895054555107,0.00549718967396158,
0.0087498394949498),.UNSPECIFIED.);
#3665=B_SPLINE_CURVE_WITH_KNOTS('',3,(#88135,#88136,#88137,#88138,#88139,
#88140,#88141),.UNSPECIFIED.,.F.,.F.,(4,3,4),(0.0010048444099522,0.00549718948033446,
0.00935178896934135),.UNSPECIFIED.);
#3666=B_SPLINE_CURVE_WITH_KNOTS('',3,(#88144,#88145,#88146,#88147,#88148,
#88149,#88150),.UNSPECIFIED.,.F.,.F.,(4,3,4),(0.000402895054555106,0.00549718967396158,
0.00874983947706886),.UNSPECIFIED.);
#3667=B_SPLINE_CURVE_WITH_KNOTS('',3,(#88155,#88156,#88157,#88158,#88159,
#88160,#88161),.UNSPECIFIED.,.F.,.F.,(4,3,4),(1.68383824729309E-5,0.00549718950318958,
0.00836378288127802),.UNSPECIFIED.);
#3668=B_SPLINE_CURVE_WITH_KNOTS('',3,(#88164,#88165,#88166,#88167,#88168,
#88169,#88170),.UNSPECIFIED.,.F.,.F.,(4,3,4),(0.000402895054555107,0.00549718967396158,
0.00874983950741581),.UNSPECIFIED.);
#3669=B_SPLINE_CURVE_WITH_KNOTS('',3,(#88175,#88176,#88177,#88178,#88179,
#88180,#88181),.UNSPECIFIED.,.F.,.F.,(4,3,4),(0.0010048444099522,0.00549718948033446,
0.00935178896934135),.UNSPECIFIED.);
#3670=B_SPLINE_CURVE_WITH_KNOTS('',3,(#88184,#88185,#88186,#88187,#88188,
#88189,#88190),.UNSPECIFIED.,.F.,.F.,(4,3,4),(0.000402895054555113,0.00549718967396158,
0.00874983950741582),.UNSPECIFIED.);
#3671=B_SPLINE_CURVE_WITH_KNOTS('',3,(#88195,#88196,#88197,#88198,#88199,
#88200,#88201),.UNSPECIFIED.,.F.,.F.,(4,3,4),(0.000117964457281399,0.00549718950073096,
0.00846490896228074),.UNSPECIFIED.);
#3672=B_SPLINE_CURVE_WITH_KNOTS('',3,(#88204,#88205,#88206,#88207,#88208,
#88209,#88210),.UNSPECIFIED.,.F.,.F.,(4,3,4),(0.000402895054555107,0.00549718967396158,
0.00874983950741581),.UNSPECIFIED.);
#3673=B_SPLINE_CURVE_WITH_KNOTS('',3,(#88215,#88216,#88217,#88218,#88219,
#88220,#88221),.UNSPECIFIED.,.F.,.F.,(4,3,4),(0.0010048444099522,0.00549718948033446,
0.00935178896934134),.UNSPECIFIED.);
#3674=B_SPLINE_CURVE_WITH_KNOTS('',3,(#88224,#88225,#88226,#88227,#88228,
#88229,#88230),.UNSPECIFIED.,.F.,.F.,(4,3,4),(0.000402895054555106,0.00549718967396158,
0.00874983948021838),.UNSPECIFIED.);
#4118=LINE('',#87735,#4588);
#4119=LINE('',#87738,#4589);
#4120=LINE('',#87747,#4590);
#4121=LINE('',#87757,#4591);
#4122=LINE('',#87774,#4592);
#4123=LINE('',#87776,#4593);
#4124=LINE('',#87779,#4594);
#4125=LINE('',#87792,#4595);
#4126=LINE('',#88006,#4596);
#4127=LINE('',#88019,#4597);
#4128=LINE('',#88337,#4598);
#4129=LINE('',#88345,#4599);
#4130=LINE('',#88349,#4600);
#4131=LINE('',#88353,#4601);
#4132=LINE('',#88356,#4602);
#4133=LINE('',#88360,#4603);
#4134=LINE('',#88367,#4604);
#4135=LINE('',#88375,#4605);
#4136=LINE('',#88383,#4606);
#4137=LINE('',#88391,#4607);
#4138=LINE('',#88399,#4608);
#4139=LINE('',#88407,#4609);
#4140=LINE('',#88415,#4610);
#4141=LINE('',#88423,#4611);
#4142=LINE('',#88431,#4612);
#4143=LINE('',#88439,#4613);
#4144=LINE('',#88447,#4614);
#4588=VECTOR('',#16822,15.4);
#4589=VECTOR('',#16827,20.);
#4590=VECTOR('',#16838,12.7058184384753);
#4591=VECTOR('',#16849,16.6071946160828);
#4592=VECTOR('',#16870,13.3064408708579);
#4593=VECTOR('',#16873,12.4591576910941);
#4594=VECTOR('',#16876,13.0685506725942);
#4595=VECTOR('',#16881,13.0685506725942);
#4596=VECTOR('',#16928,17.5762965073726);
#4597=VECTOR('',#16933,17.5762965073726);
#4598=VECTOR('',#17176,10.6410293263727);
#4599=VECTOR('',#17185,12.6998790237181);
#4600=VECTOR('',#17190,14.0317131491268);
#4601=VECTOR('',#17195,14.0317131491268);
#4602=VECTOR('',#17200,8.5);
#4603=VECTOR('',#17205,11.9728634517814);
#4604=VECTOR('',#17214,2.62159462638384);
#4605=VECTOR('',#17225,2.62159462638384);
#4606=VECTOR('',#17236,2.62159462638384);
#4607=VECTOR('',#17247,2.62159462638384);
#4608=VECTOR('',#17258,2.62159462638384);
#4609=VECTOR('',#17269,2.62159462638384);
#4610=VECTOR('',#17280,2.62159462638384);
#4611=VECTOR('',#17291,2.62159462638384);
#4612=VECTOR('',#17302,2.62159462638384);
#4613=VECTOR('',#17313,2.62159462638384);
#4614=VECTOR('',#17324,2.62159462638384);
#5901=VERTEX_POINT('',#87718);
#5902=VERTEX_POINT('',#87719);
#5903=VERTEX_POINT('',#87722);
#5904=VERTEX_POINT('',#87726);
#5905=VERTEX_POINT('',#87728);
#5906=VERTEX_POINT('',#87732);
#5907=VERTEX_POINT('',#87734);
#5908=VERTEX_POINT('',#87742);
#5909=VERTEX_POINT('',#87743);
#5910=VERTEX_POINT('',#87746);
#5911=VERTEX_POINT('',#87748);
#5912=VERTEX_POINT('',#87752);
#5913=VERTEX_POINT('',#87753);
#5914=VERTEX_POINT('',#87756);
#5915=VERTEX_POINT('',#87758);
#5916=VERTEX_POINT('',#87762);
#5917=VERTEX_POINT('',#87764);
#5918=VERTEX_POINT('',#87766);
#5919=VERTEX_POINT('',#87770);
#5920=VERTEX_POINT('',#87771);
#5921=VERTEX_POINT('',#87778);
#5922=VERTEX_POINT('',#87780);
#5923=VERTEX_POINT('',#87782);
#5924=VERTEX_POINT('',#87790);
#5925=VERTEX_POINT('',#87793);
#5926=VERTEX_POINT('',#87795);
#5927=VERTEX_POINT('',#87804);
#5928=VERTEX_POINT('',#87805);
#5929=VERTEX_POINT('',#87807);
#5930=VERTEX_POINT('',#87815);
#5931=VERTEX_POINT('',#87824);
#5932=VERTEX_POINT('',#87825);
#5933=VERTEX_POINT('',#87827);
#5934=VERTEX_POINT('',#87835);
#5935=VERTEX_POINT('',#87844);
#5936=VERTEX_POINT('',#87845);
#5937=VERTEX_POINT('',#87847);
#5938=VERTEX_POINT('',#87855);
#5939=VERTEX_POINT('',#87864);
#5940=VERTEX_POINT('',#87865);
#5941=VERTEX_POINT('',#87867);
#5942=VERTEX_POINT('',#87875);
#5943=VERTEX_POINT('',#87884);
#5944=VERTEX_POINT('',#87885);
#5945=VERTEX_POINT('',#87887);
#5946=VERTEX_POINT('',#87895);
#5947=VERTEX_POINT('',#87904);
#5948=VERTEX_POINT('',#87905);
#5949=VERTEX_POINT('',#87907);
#5950=VERTEX_POINT('',#87915);
#5951=VERTEX_POINT('',#87924);
#5952=VERTEX_POINT('',#87925);
#5953=VERTEX_POINT('',#87927);
#5954=VERTEX_POINT('',#87935);
#5955=VERTEX_POINT('',#87944);
#5956=VERTEX_POINT('',#87945);
#5957=VERTEX_POINT('',#87947);
#5958=VERTEX_POINT('',#87955);
#5959=VERTEX_POINT('',#87964);
#5960=VERTEX_POINT('',#87965);
#5961=VERTEX_POINT('',#87967);
#5962=VERTEX_POINT('',#87975);
#5963=VERTEX_POINT('',#87984);
#5964=VERTEX_POINT('',#87985);
#5965=VERTEX_POINT('',#87987);
#5966=VERTEX_POINT('',#87995);
#5967=VERTEX_POINT('',#88005);
#5968=VERTEX_POINT('',#88007);
#5969=VERTEX_POINT('',#88009);
#5970=VERTEX_POINT('',#88017);
#5971=VERTEX_POINT('',#88020);
#5972=VERTEX_POINT('',#88022);
#5973=VERTEX_POINT('',#88031);
#5974=VERTEX_POINT('',#88032);
#5975=VERTEX_POINT('',#88034);
#5976=VERTEX_POINT('',#88042);
#5977=VERTEX_POINT('',#88051);
#5978=VERTEX_POINT('',#88052);
#5979=VERTEX_POINT('',#88054);
#5980=VERTEX_POINT('',#88062);
#5981=VERTEX_POINT('',#88071);
#5982=VERTEX_POINT('',#88072);
#5983=VERTEX_POINT('',#88074);
#5984=VERTEX_POINT('',#88082);
#5985=VERTEX_POINT('',#88091);
#5986=VERTEX_POINT('',#88092);
#5987=VERTEX_POINT('',#88094);
#5988=VERTEX_POINT('',#88102);
#5989=VERTEX_POINT('',#88111);
#5990=VERTEX_POINT('',#88112);
#5991=VERTEX_POINT('',#88114);
#5992=VERTEX_POINT('',#88122);
#5993=VERTEX_POINT('',#88131);
#5994=VERTEX_POINT('',#88132);
#5995=VERTEX_POINT('',#88134);
#5996=VERTEX_POINT('',#88142);
#5997=VERTEX_POINT('',#88151);
#5998=VERTEX_POINT('',#88152);
#5999=VERTEX_POINT('',#88154);
#6000=VERTEX_POINT('',#88162);
#6001=VERTEX_POINT('',#88171);
#6002=VERTEX_POINT('',#88172);
#6003=VERTEX_POINT('',#88174);
#6004=VERTEX_POINT('',#88182);
#6005=VERTEX_POINT('',#88191);
#6006=VERTEX_POINT('',#88192);
#6007=VERTEX_POINT('',#88194);
#6008=VERTEX_POINT('',#88202);
#6009=VERTEX_POINT('',#88211);
#6010=VERTEX_POINT('',#88212);
#6011=VERTEX_POINT('',#88214);
#6012=VERTEX_POINT('',#88222);
#6013=VERTEX_POINT('',#88320);
#6014=VERTEX_POINT('',#88322);
#6015=VERTEX_POINT('',#88324);
#6016=VERTEX_POINT('',#88328);
#6017=VERTEX_POINT('',#88330);
#6018=VERTEX_POINT('',#88334);
#6019=VERTEX_POINT('',#88336);
#6020=VERTEX_POINT('',#88338);
#6021=VERTEX_POINT('',#88342);
#6022=VERTEX_POINT('',#88343);
#6023=VERTEX_POINT('',#88348);
#6024=VERTEX_POINT('',#88352);
#6025=VERTEX_POINT('',#88358);
#6026=VERTEX_POINT('',#88364);
#6027=VERTEX_POINT('',#88366);
#6028=VERTEX_POINT('',#88372);
#6029=VERTEX_POINT('',#88374);
#6030=VERTEX_POINT('',#88380);
#6031=VERTEX_POINT('',#88382);
#6032=VERTEX_POINT('',#88388);
#6033=VERTEX_POINT('',#88390);
#6034=VERTEX_POINT('',#88396);
#6035=VERTEX_POINT('',#88398);
#6036=VERTEX_POINT('',#88404);
#6037=VERTEX_POINT('',#88406);
#6038=VERTEX_POINT('',#88412);
#6039=VERTEX_POINT('',#88414);
#6040=VERTEX_POINT('',#88420);
#6041=VERTEX_POINT('',#88422);
#6042=VERTEX_POINT('',#88428);
#6043=VERTEX_POINT('',#88430);
#6044=VERTEX_POINT('',#88436);
#6045=VERTEX_POINT('',#88438);
#6046=VERTEX_POINT('',#88444);
#6047=VERTEX_POINT('',#88446);
#7849=EDGE_CURVE('',#5901,#5902,#2768,.T.);
#7850=EDGE_CURVE('',#5902,#5901,#2769,.T.);
#7851=EDGE_CURVE('',#5902,#5903,#2770,.T.);
#7852=EDGE_CURVE('',#5903,#5903,#2771,.T.);
#7853=EDGE_CURVE('',#5904,#5904,#2772,.T.);
#7854=EDGE_CURVE('',#5904,#5905,#2773,.T.);
#7855=EDGE_CURVE('',#5905,#5905,#2774,.T.);
#7856=EDGE_CURVE('',#5906,#5906,#2775,.T.);
#7857=EDGE_CURVE('',#5906,#5907,#4118,.T.);
#7858=EDGE_CURVE('',#5907,#5907,#2776,.T.);
#7859=EDGE_CURVE('',#5901,#5904,#4119,.T.);
#7860=EDGE_CURVE('',#5908,#5909,#2777,.T.);
#7861=EDGE_CURVE('',#5909,#5908,#2778,.T.);
#7862=EDGE_CURVE('',#5909,#5910,#4120,.T.);
#7863=EDGE_CURVE('',#5910,#5911,#2779,.T.);
#7864=EDGE_CURVE('',#5911,#5910,#2780,.T.);
#7865=EDGE_CURVE('',#5912,#5913,#2781,.T.);
#7866=EDGE_CURVE('',#5913,#5912,#2782,.T.);
#7867=EDGE_CURVE('',#5913,#5914,#4121,.T.);
#7868=EDGE_CURVE('',#5914,#5915,#2783,.T.);
#7869=EDGE_CURVE('',#5915,#5914,#2784,.T.);
#7870=EDGE_CURVE('',#5916,#5916,#2785,.T.);
#7871=EDGE_CURVE('',#5916,#5917,#2786,.T.);
#7872=EDGE_CURVE('',#5917,#5918,#2787,.T.);
#7873=EDGE_CURVE('',#5918,#5917,#2788,.T.);
#7874=EDGE_CURVE('',#5919,#5920,#2789,.T.);
#7875=EDGE_CURVE('',#5920,#5919,#2790,.T.);
#7876=EDGE_CURVE('',#5920,#5916,#4122,.T.);
#7877=EDGE_CURVE('',#5919,#5911,#4123,.T.);
#7878=EDGE_CURVE('',#5908,#5921,#4124,.T.);
#7879=EDGE_CURVE('',#5921,#5922,#242,.T.);
#7880=EDGE_CURVE('',#5922,#5923,#3631,.T.);
#7881=EDGE_CURVE('',#5924,#5923,#243,.T.);
#7882=EDGE_CURVE('',#5924,#5915,#4125,.T.);
#7883=EDGE_CURVE('',#5925,#5924,#244,.T.);
#7884=EDGE_CURVE('',#5925,#5926,#3632,.T.);
#7885=EDGE_CURVE('',#5926,#5921,#245,.T.);
#7886=EDGE_CURVE('',#5927,#5928,#246,.F.);
#7887=EDGE_CURVE('',#5928,#5929,#3633,.T.);
#7888=EDGE_CURVE('',#5930,#5929,#247,.F.);
#7889=EDGE_CURVE('',#5930,#5927,#3634,.T.);
#7890=EDGE_CURVE('',#5931,#5932,#248,.T.);
#7891=EDGE_CURVE('',#5931,#5933,#3635,.T.);
#7892=EDGE_CURVE('',#5933,#5934,#249,.T.);
#7893=EDGE_CURVE('',#5934,#5932,#3636,.T.);
#7894=EDGE_CURVE('',#5935,#5936,#250,.T.);
#7895=EDGE_CURVE('',#5935,#5937,#3637,.T.);
#7896=EDGE_CURVE('',#5937,#5938,#251,.T.);
#7897=EDGE_CURVE('',#5938,#5936,#3638,.T.);
#7898=EDGE_CURVE('',#5939,#5940,#252,.T.);
#7899=EDGE_CURVE('',#5939,#5941,#3639,.T.);
#7900=EDGE_CURVE('',#5941,#5942,#253,.T.);
#7901=EDGE_CURVE('',#5942,#5940,#3640,.T.);
#7902=EDGE_CURVE('',#5943,#5944,#254,.T.);
#7903=EDGE_CURVE('',#5943,#5945,#3641,.T.);
#7904=EDGE_CURVE('',#5945,#5946,#255,.T.);
#7905=EDGE_CURVE('',#5946,#5944,#3642,.T.);
#7906=EDGE_CURVE('',#5947,#5948,#256,.T.);
#7907=EDGE_CURVE('',#5947,#5949,#3643,.T.);
#7908=EDGE_CURVE('',#5949,#5950,#257,.T.);
#7909=EDGE_CURVE('',#5950,#5948,#3644,.T.);
#7910=EDGE_CURVE('',#5951,#5952,#258,.T.);
#7911=EDGE_CURVE('',#5951,#5953,#3645,.T.);
#7912=EDGE_CURVE('',#5953,#5954,#259,.T.);
#7913=EDGE_CURVE('',#5954,#5952,#3646,.T.);
#7914=EDGE_CURVE('',#5955,#5956,#260,.T.);
#7915=EDGE_CURVE('',#5955,#5957,#3647,.T.);
#7916=EDGE_CURVE('',#5957,#5958,#261,.T.);
#7917=EDGE_CURVE('',#5958,#5956,#3648,.T.);
#7918=EDGE_CURVE('',#5959,#5960,#262,.T.);
#7919=EDGE_CURVE('',#5959,#5961,#3649,.T.);
#7920=EDGE_CURVE('',#5961,#5962,#263,.T.);
#7921=EDGE_CURVE('',#5962,#5960,#3650,.T.);
#7922=EDGE_CURVE('',#5963,#5964,#264,.T.);
#7923=EDGE_CURVE('',#5963,#5965,#3651,.T.);
#7924=EDGE_CURVE('',#5965,#5966,#265,.T.);
#7925=EDGE_CURVE('',#5966,#5964,#3652,.T.);
#7926=EDGE_CURVE('',#5912,#5967,#4126,.T.);
#7927=EDGE_CURVE('',#5968,#5967,#266,.T.);
#7928=EDGE_CURVE('',#5968,#5969,#3653,.T.);
#7929=EDGE_CURVE('',#5969,#5970,#267,.T.);
#7930=EDGE_CURVE('',#5970,#5918,#4127,.T.);
#7931=EDGE_CURVE('',#5970,#5971,#268,.T.);
#7932=EDGE_CURVE('',#5971,#5972,#3654,.T.);
#7933=EDGE_CURVE('',#5967,#5972,#269,.T.);
#7934=EDGE_CURVE('',#5973,#5974,#270,.F.);
#7935=EDGE_CURVE('',#5974,#5975,#3655,.T.);
#7936=EDGE_CURVE('',#5976,#5975,#271,.F.);
#7937=EDGE_CURVE('',#5976,#5973,#3656,.T.);
#7938=EDGE_CURVE('',#5977,#5978,#272,.T.);
#7939=EDGE_CURVE('',#5977,#5979,#3657,.T.);
#7940=EDGE_CURVE('',#5979,#5980,#273,.T.);
#7941=EDGE_CURVE('',#5980,#5978,#3658,.T.);
#7942=EDGE_CURVE('',#5981,#5982,#274,.T.);
#7943=EDGE_CURVE('',#5981,#5983,#3659,.T.);
#7944=EDGE_CURVE('',#5983,#5984,#275,.T.);
#7945=EDGE_CURVE('',#5984,#5982,#3660,.T.);
#7946=EDGE_CURVE('',#5985,#5986,#276,.T.);
#7947=EDGE_CURVE('',#5985,#5987,#3661,.T.);
#7948=EDGE_CURVE('',#5987,#5988,#277,.T.);
#7949=EDGE_CURVE('',#5988,#5986,#3662,.T.);
#7950=EDGE_CURVE('',#5989,#5990,#278,.T.);
#7951=EDGE_CURVE('',#5989,#5991,#3663,.T.);
#7952=EDGE_CURVE('',#5991,#5992,#279,.T.);
#7953=EDGE_CURVE('',#5992,#5990,#3664,.T.);
#7954=EDGE_CURVE('',#5993,#5994,#280,.T.);
#7955=EDGE_CURVE('',#5993,#5995,#3665,.T.);
#7956=EDGE_CURVE('',#5995,#5996,#281,.T.);
#7957=EDGE_CURVE('',#5996,#5994,#3666,.T.);
#7958=EDGE_CURVE('',#5997,#5998,#282,.T.);
#7959=EDGE_CURVE('',#5997,#5999,#3667,.T.);
#7960=EDGE_CURVE('',#5999,#6000,#283,.T.);
#7961=EDGE_CURVE('',#6000,#5998,#3668,.T.);
#7962=EDGE_CURVE('',#6001,#6002,#284,.T.);
#7963=EDGE_CURVE('',#6001,#6003,#3669,.T.);
#7964=EDGE_CURVE('',#6003,#6004,#285,.T.);
#7965=EDGE_CURVE('',#6004,#6002,#3670,.T.);
#7966=EDGE_CURVE('',#6005,#6006,#286,.T.);
#7967=EDGE_CURVE('',#6005,#6007,#3671,.T.);
#7968=EDGE_CURVE('',#6007,#6008,#287,.T.);
#7969=EDGE_CURVE('',#6008,#6006,#3672,.T.);
#7970=EDGE_CURVE('',#6009,#6010,#288,.T.);
#7971=EDGE_CURVE('',#6009,#6011,#3673,.T.);
#7972=EDGE_CURVE('',#6011,#6012,#289,.T.);
#7973=EDGE_CURVE('',#6012,#6010,#3674,.T.);
#7974=EDGE_CURVE('',#6004,#5941,#2791,.T.);
#7975=EDGE_CURVE('',#6002,#5939,#2792,.T.);
#7976=EDGE_CURVE('',#5940,#6001,#2793,.T.);
#7977=EDGE_CURVE('',#5942,#6003,#2794,.T.);
#7978=EDGE_CURVE('',#6008,#5945,#2795,.T.);
#7979=EDGE_CURVE('',#6006,#5943,#2796,.T.);
#7980=EDGE_CURVE('',#5944,#6005,#2797,.T.);
#7981=EDGE_CURVE('',#5946,#6007,#2798,.T.);
#7982=EDGE_CURVE('',#6000,#5937,#2799,.T.);
#7983=EDGE_CURVE('',#5998,#5935,#2800,.T.);
#7984=EDGE_CURVE('',#5936,#5997,#2801,.T.);
#7985=EDGE_CURVE('',#5938,#5999,#2802,.T.);
#7986=EDGE_CURVE('',#6012,#5949,#2803,.T.);
#7987=EDGE_CURVE('',#6010,#5947,#2804,.T.);
#7988=EDGE_CURVE('',#5948,#6009,#2805,.T.);
#7989=EDGE_CURVE('',#5950,#6011,#2806,.T.);
#7990=EDGE_CURVE('',#5974,#5927,#2807,.T.);
#7991=EDGE_CURVE('',#5975,#5930,#2808,.T.);
#7992=EDGE_CURVE('',#5929,#5976,#2809,.T.);
#7993=EDGE_CURVE('',#5928,#5973,#2810,.T.);
#7994=EDGE_CURVE('',#5988,#5961,#2811,.T.);
#7995=EDGE_CURVE('',#5986,#5959,#2812,.T.);
#7996=EDGE_CURVE('',#5960,#5985,#2813,.T.);
#7997=EDGE_CURVE('',#5962,#5987,#2814,.T.);
#7998=EDGE_CURVE('',#5984,#5957,#2815,.T.);
#7999=EDGE_CURVE('',#5982,#5955,#2816,.T.);
#8000=EDGE_CURVE('',#5956,#5981,#2817,.T.);
#8001=EDGE_CURVE('',#5958,#5983,#2818,.T.);
#8002=EDGE_CURVE('',#5992,#5965,#2819,.T.);
#8003=EDGE_CURVE('',#5990,#5963,#2820,.T.);
#8004=EDGE_CURVE('',#5964,#5989,#2821,.T.);
#8005=EDGE_CURVE('',#5966,#5991,#2822,.T.);
#8006=EDGE_CURVE('',#5980,#5953,#2823,.T.);
#8007=EDGE_CURVE('',#5978,#5951,#2824,.T.);
#8008=EDGE_CURVE('',#5952,#5977,#2825,.T.);
#8009=EDGE_CURVE('',#5954,#5979,#2826,.T.);
#8010=EDGE_CURVE('',#5971,#5926,#2827,.T.);
#8011=EDGE_CURVE('',#5972,#5925,#2828,.T.);
#8012=EDGE_CURVE('',#5923,#5968,#2829,.T.);
#8013=EDGE_CURVE('',#5922,#5969,#2830,.T.);
#8014=EDGE_CURVE('',#5996,#5933,#2831,.T.);
#8015=EDGE_CURVE('',#5994,#5931,#2832,.T.);
#8016=EDGE_CURVE('',#5932,#5993,#2833,.T.);
#8017=EDGE_CURVE('',#5934,#5995,#2834,.T.);
#8018=EDGE_CURVE('',#6013,#6013,#2835,.T.);
#8019=EDGE_CURVE('',#6013,#6014,#2836,.T.);
#8020=EDGE_CURVE('',#6015,#6014,#2837,.T.);
#8021=EDGE_CURVE('',#6014,#6015,#2838,.T.);
#8022=EDGE_CURVE('',#6016,#6016,#2839,.T.);
#8023=EDGE_CURVE('',#6016,#6017,#2840,.T.);
#8024=EDGE_CURVE('',#6017,#6017,#2841,.T.);
#8025=EDGE_CURVE('',#6018,#6018,#2842,.T.);
#8026=EDGE_CURVE('',#6018,#6019,#4128,.T.);
#8027=EDGE_CURVE('',#6019,#6020,#2843,.T.);
#8028=EDGE_CURVE('',#6020,#6019,#2844,.T.);
#8029=EDGE_CURVE('',#6021,#6022,#2845,.T.);
#8030=EDGE_CURVE('',#6022,#6020,#4129,.T.);
#8031=EDGE_CURVE('',#6022,#6021,#2846,.T.);
#8032=EDGE_CURVE('',#6021,#6023,#4130,.T.);
#8033=EDGE_CURVE('',#6023,#6023,#2847,.T.);
#8034=EDGE_CURVE('',#6023,#6024,#4131,.T.);
#8035=EDGE_CURVE('',#6024,#6024,#2848,.T.);
#8036=EDGE_CURVE('',#6017,#6015,#4132,.T.);
#8037=EDGE_CURVE('',#6025,#6025,#2849,.T.);
#8038=EDGE_CURVE('',#6025,#6018,#4133,.T.);
#8039=EDGE_CURVE('',#6026,#6026,#2850,.T.);
#8040=EDGE_CURVE('',#6026,#6027,#4134,.T.);
#8041=EDGE_CURVE('',#6027,#6027,#2851,.T.);
#8042=EDGE_CURVE('',#6028,#6028,#2852,.T.);
#8043=EDGE_CURVE('',#6028,#6029,#4135,.T.);
#8044=EDGE_CURVE('',#6029,#6029,#2853,.T.);
#8045=EDGE_CURVE('',#6030,#6030,#2854,.T.);
#8046=EDGE_CURVE('',#6030,#6031,#4136,.T.);
#8047=EDGE_CURVE('',#6031,#6031,#2855,.T.);
#8048=EDGE_CURVE('',#6032,#6032,#2856,.T.);
#8049=EDGE_CURVE('',#6032,#6033,#4137,.T.);
#8050=EDGE_CURVE('',#6033,#6033,#2857,.T.);
#8051=EDGE_CURVE('',#6034,#6034,#2858,.T.);
#8052=EDGE_CURVE('',#6034,#6035,#4138,.T.);
#8053=EDGE_CURVE('',#6035,#6035,#2859,.T.);
#8054=EDGE_CURVE('',#6036,#6036,#2860,.T.);
#8055=EDGE_CURVE('',#6036,#6037,#4139,.T.);
#8056=EDGE_CURVE('',#6037,#6037,#2861,.T.);
#8057=EDGE_CURVE('',#6038,#6038,#2862,.T.);
#8058=EDGE_CURVE('',#6038,#6039,#4140,.T.);
#8059=EDGE_CURVE('',#6039,#6039,#2863,.T.);
#8060=EDGE_CURVE('',#6040,#6040,#2864,.T.);
#8061=EDGE_CURVE('',#6040,#6041,#4141,.T.);
#8062=EDGE_CURVE('',#6041,#6041,#2865,.T.);
#8063=EDGE_CURVE('',#6042,#6042,#2866,.T.);
#8064=EDGE_CURVE('',#6042,#6043,#4142,.T.);
#8065=EDGE_CURVE('',#6043,#6043,#2867,.T.);
#8066=EDGE_CURVE('',#6044,#6044,#2868,.T.);
#8067=EDGE_CURVE('',#6044,#6045,#4143,.T.);
#8068=EDGE_CURVE('',#6045,#6045,#2869,.T.);
#8069=EDGE_CURVE('',#6046,#6046,#2870,.T.);
#8070=EDGE_CURVE('',#6046,#6047,#4144,.T.);
#8071=EDGE_CURVE('',#6047,#6047,#2871,.T.);
#11674=ORIENTED_EDGE('',*,*,#7849,.F.);
#11675=ORIENTED_EDGE('',*,*,#7850,.F.);
#11676=ORIENTED_EDGE('',*,*,#7851,.T.);
#11677=ORIENTED_EDGE('',*,*,#7852,.F.);
#11678=ORIENTED_EDGE('',*,*,#7851,.F.);
#11679=ORIENTED_EDGE('',*,*,#7853,.F.);
#11680=ORIENTED_EDGE('',*,*,#7854,.T.);
#11681=ORIENTED_EDGE('',*,*,#7855,.F.);
#11682=ORIENTED_EDGE('',*,*,#7854,.F.);
#11683=ORIENTED_EDGE('',*,*,#7856,.T.);
#11684=ORIENTED_EDGE('',*,*,#7857,.T.);
#11685=ORIENTED_EDGE('',*,*,#7858,.F.);
#11686=ORIENTED_EDGE('',*,*,#7857,.F.);
#11687=ORIENTED_EDGE('',*,*,#7849,.T.);
#11688=ORIENTED_EDGE('',*,*,#7850,.T.);
#11689=ORIENTED_EDGE('',*,*,#7859,.T.);
#11690=ORIENTED_EDGE('',*,*,#7853,.T.);
#11691=ORIENTED_EDGE('',*,*,#7859,.F.);
#11692=ORIENTED_EDGE('',*,*,#7852,.T.);
#11693=ORIENTED_EDGE('',*,*,#7856,.F.);
#11694=ORIENTED_EDGE('',*,*,#7855,.T.);
#11695=ORIENTED_EDGE('',*,*,#7858,.T.);
#11696=ORIENTED_EDGE('',*,*,#7860,.F.);
#11697=ORIENTED_EDGE('',*,*,#7861,.F.);
#11698=ORIENTED_EDGE('',*,*,#7862,.T.);
#11699=ORIENTED_EDGE('',*,*,#7863,.T.);
#11700=ORIENTED_EDGE('',*,*,#7864,.T.);
#11701=ORIENTED_EDGE('',*,*,#7862,.F.);
#11702=ORIENTED_EDGE('',*,*,#7865,.F.);
#11703=ORIENTED_EDGE('',*,*,#7866,.F.);
#11704=ORIENTED_EDGE('',*,*,#7867,.T.);
#11705=ORIENTED_EDGE('',*,*,#7868,.T.);
#11706=ORIENTED_EDGE('',*,*,#7869,.T.);
#11707=ORIENTED_EDGE('',*,*,#7867,.F.);
#11708=ORIENTED_EDGE('',*,*,#7870,.F.);
#11709=ORIENTED_EDGE('',*,*,#7871,.T.);
#11710=ORIENTED_EDGE('',*,*,#7872,.T.);
#11711=ORIENTED_EDGE('',*,*,#7873,.T.);
#11712=ORIENTED_EDGE('',*,*,#7871,.F.);
#11713=ORIENTED_EDGE('',*,*,#7874,.F.);
#11714=ORIENTED_EDGE('',*,*,#7875,.F.);
#11715=ORIENTED_EDGE('',*,*,#7876,.T.);
#11716=ORIENTED_EDGE('',*,*,#7870,.T.);
#11717=ORIENTED_EDGE('',*,*,#7876,.F.);
#11718=ORIENTED_EDGE('',*,*,#7874,.T.);
#11719=ORIENTED_EDGE('',*,*,#7875,.T.);
#11720=ORIENTED_EDGE('',*,*,#7877,.T.);
#11721=ORIENTED_EDGE('',*,*,#7863,.F.);
#11722=ORIENTED_EDGE('',*,*,#7864,.F.);
#11723=ORIENTED_EDGE('',*,*,#7877,.F.);
#11724=ORIENTED_EDGE('',*,*,#7860,.T.);
#11725=ORIENTED_EDGE('',*,*,#7861,.T.);
#11726=ORIENTED_EDGE('',*,*,#7878,.T.);
#11727=ORIENTED_EDGE('',*,*,#7879,.T.);
#11728=ORIENTED_EDGE('',*,*,#7880,.T.);
#11729=ORIENTED_EDGE('',*,*,#7881,.F.);
#11730=ORIENTED_EDGE('',*,*,#7882,.T.);
#11731=ORIENTED_EDGE('',*,*,#7868,.F.);
#11732=ORIENTED_EDGE('',*,*,#7869,.F.);
#11733=ORIENTED_EDGE('',*,*,#7882,.F.);
#11734=ORIENTED_EDGE('',*,*,#7883,.F.);
#11735=ORIENTED_EDGE('',*,*,#7884,.T.);
#11736=ORIENTED_EDGE('',*,*,#7885,.T.);
#11737=ORIENTED_EDGE('',*,*,#7878,.F.);
#11738=ORIENTED_EDGE('',*,*,#7886,.T.);
#11739=ORIENTED_EDGE('',*,*,#7887,.T.);
#11740=ORIENTED_EDGE('',*,*,#7888,.F.);
#11741=ORIENTED_EDGE('',*,*,#7889,.T.);
#11742=ORIENTED_EDGE('',*,*,#7890,.F.);
#11743=ORIENTED_EDGE('',*,*,#7891,.T.);
#11744=ORIENTED_EDGE('',*,*,#7892,.T.);
#11745=ORIENTED_EDGE('',*,*,#7893,.T.);
#11746=ORIENTED_EDGE('',*,*,#7894,.F.);
#11747=ORIENTED_EDGE('',*,*,#7895,.T.);
#11748=ORIENTED_EDGE('',*,*,#7896,.T.);
#11749=ORIENTED_EDGE('',*,*,#7897,.T.);
#11750=ORIENTED_EDGE('',*,*,#7898,.F.);
#11751=ORIENTED_EDGE('',*,*,#7899,.T.);
#11752=ORIENTED_EDGE('',*,*,#7900,.T.);
#11753=ORIENTED_EDGE('',*,*,#7901,.T.);
#11754=ORIENTED_EDGE('',*,*,#7902,.F.);
#11755=ORIENTED_EDGE('',*,*,#7903,.T.);
#11756=ORIENTED_EDGE('',*,*,#7904,.T.);
#11757=ORIENTED_EDGE('',*,*,#7905,.T.);
#11758=ORIENTED_EDGE('',*,*,#7906,.F.);
#11759=ORIENTED_EDGE('',*,*,#7907,.T.);
#11760=ORIENTED_EDGE('',*,*,#7908,.T.);
#11761=ORIENTED_EDGE('',*,*,#7909,.T.);
#11762=ORIENTED_EDGE('',*,*,#7910,.F.);
#11763=ORIENTED_EDGE('',*,*,#7911,.T.);
#11764=ORIENTED_EDGE('',*,*,#7912,.T.);
#11765=ORIENTED_EDGE('',*,*,#7913,.T.);
#11766=ORIENTED_EDGE('',*,*,#7914,.F.);
#11767=ORIENTED_EDGE('',*,*,#7915,.T.);
#11768=ORIENTED_EDGE('',*,*,#7916,.T.);
#11769=ORIENTED_EDGE('',*,*,#7917,.T.);
#11770=ORIENTED_EDGE('',*,*,#7918,.F.);
#11771=ORIENTED_EDGE('',*,*,#7919,.T.);
#11772=ORIENTED_EDGE('',*,*,#7920,.T.);
#11773=ORIENTED_EDGE('',*,*,#7921,.T.);
#11774=ORIENTED_EDGE('',*,*,#7922,.F.);
#11775=ORIENTED_EDGE('',*,*,#7923,.T.);
#11776=ORIENTED_EDGE('',*,*,#7924,.T.);
#11777=ORIENTED_EDGE('',*,*,#7925,.T.);
#11778=ORIENTED_EDGE('',*,*,#7865,.T.);
#11779=ORIENTED_EDGE('',*,*,#7866,.T.);
#11780=ORIENTED_EDGE('',*,*,#7926,.T.);
#11781=ORIENTED_EDGE('',*,*,#7927,.F.);
#11782=ORIENTED_EDGE('',*,*,#7928,.T.);
#11783=ORIENTED_EDGE('',*,*,#7929,.T.);
#11784=ORIENTED_EDGE('',*,*,#7930,.T.);
#11785=ORIENTED_EDGE('',*,*,#7872,.F.);
#11786=ORIENTED_EDGE('',*,*,#7873,.F.);
#11787=ORIENTED_EDGE('',*,*,#7930,.F.);
#11788=ORIENTED_EDGE('',*,*,#7931,.T.);
#11789=ORIENTED_EDGE('',*,*,#7932,.T.);
#11790=ORIENTED_EDGE('',*,*,#7933,.F.);
#11791=ORIENTED_EDGE('',*,*,#7926,.F.);
#11792=ORIENTED_EDGE('',*,*,#7934,.T.);
#11793=ORIENTED_EDGE('',*,*,#7935,.T.);
#11794=ORIENTED_EDGE('',*,*,#7936,.F.);
#11795=ORIENTED_EDGE('',*,*,#7937,.T.);
#11796=ORIENTED_EDGE('',*,*,#7938,.F.);
#11797=ORIENTED_EDGE('',*,*,#7939,.T.);
#11798=ORIENTED_EDGE('',*,*,#7940,.T.);
#11799=ORIENTED_EDGE('',*,*,#7941,.T.);
#11800=ORIENTED_EDGE('',*,*,#7942,.F.);
#11801=ORIENTED_EDGE('',*,*,#7943,.T.);
#11802=ORIENTED_EDGE('',*,*,#7944,.T.);
#11803=ORIENTED_EDGE('',*,*,#7945,.T.);
#11804=ORIENTED_EDGE('',*,*,#7946,.F.);
#11805=ORIENTED_EDGE('',*,*,#7947,.T.);
#11806=ORIENTED_EDGE('',*,*,#7948,.T.);
#11807=ORIENTED_EDGE('',*,*,#7949,.T.);
#11808=ORIENTED_EDGE('',*,*,#7950,.F.);
#11809=ORIENTED_EDGE('',*,*,#7951,.T.);
#11810=ORIENTED_EDGE('',*,*,#7952,.T.);
#11811=ORIENTED_EDGE('',*,*,#7953,.T.);
#11812=ORIENTED_EDGE('',*,*,#7954,.F.);
#11813=ORIENTED_EDGE('',*,*,#7955,.T.);
#11814=ORIENTED_EDGE('',*,*,#7956,.T.);
#11815=ORIENTED_EDGE('',*,*,#7957,.T.);
#11816=ORIENTED_EDGE('',*,*,#7958,.F.);
#11817=ORIENTED_EDGE('',*,*,#7959,.T.);
#11818=ORIENTED_EDGE('',*,*,#7960,.T.);
#11819=ORIENTED_EDGE('',*,*,#7961,.T.);
#11820=ORIENTED_EDGE('',*,*,#7962,.F.);
#11821=ORIENTED_EDGE('',*,*,#7963,.T.);
#11822=ORIENTED_EDGE('',*,*,#7964,.T.);
#11823=ORIENTED_EDGE('',*,*,#7965,.T.);
#11824=ORIENTED_EDGE('',*,*,#7966,.F.);
#11825=ORIENTED_EDGE('',*,*,#7967,.T.);
#11826=ORIENTED_EDGE('',*,*,#7968,.T.);
#11827=ORIENTED_EDGE('',*,*,#7969,.T.);
#11828=ORIENTED_EDGE('',*,*,#7970,.F.);
#11829=ORIENTED_EDGE('',*,*,#7971,.T.);
#11830=ORIENTED_EDGE('',*,*,#7972,.T.);
#11831=ORIENTED_EDGE('',*,*,#7973,.T.);
#11832=ORIENTED_EDGE('',*,*,#7974,.T.);
#11833=ORIENTED_EDGE('',*,*,#7899,.F.);
#11834=ORIENTED_EDGE('',*,*,#7975,.F.);
#11835=ORIENTED_EDGE('',*,*,#7965,.F.);
#11836=ORIENTED_EDGE('',*,*,#7976,.F.);
#11837=ORIENTED_EDGE('',*,*,#7901,.F.);
#11838=ORIENTED_EDGE('',*,*,#7977,.T.);
#11839=ORIENTED_EDGE('',*,*,#7963,.F.);
#11840=ORIENTED_EDGE('',*,*,#7962,.T.);
#11841=ORIENTED_EDGE('',*,*,#7975,.T.);
#11842=ORIENTED_EDGE('',*,*,#7898,.T.);
#11843=ORIENTED_EDGE('',*,*,#7976,.T.);
#11844=ORIENTED_EDGE('',*,*,#7977,.F.);
#11845=ORIENTED_EDGE('',*,*,#7900,.F.);
#11846=ORIENTED_EDGE('',*,*,#7974,.F.);
#11847=ORIENTED_EDGE('',*,*,#7964,.F.);
#11848=ORIENTED_EDGE('',*,*,#7978,.T.);
#11849=ORIENTED_EDGE('',*,*,#7903,.F.);
#11850=ORIENTED_EDGE('',*,*,#7979,.F.);
#11851=ORIENTED_EDGE('',*,*,#7969,.F.);
#11852=ORIENTED_EDGE('',*,*,#7980,.F.);
#11853=ORIENTED_EDGE('',*,*,#7905,.F.);
#11854=ORIENTED_EDGE('',*,*,#7981,.T.);
#11855=ORIENTED_EDGE('',*,*,#7967,.F.);
#11856=ORIENTED_EDGE('',*,*,#7966,.T.);
#11857=ORIENTED_EDGE('',*,*,#7979,.T.);
#11858=ORIENTED_EDGE('',*,*,#7902,.T.);
#11859=ORIENTED_EDGE('',*,*,#7980,.T.);
#11860=ORIENTED_EDGE('',*,*,#7981,.F.);
#11861=ORIENTED_EDGE('',*,*,#7904,.F.);
#11862=ORIENTED_EDGE('',*,*,#7978,.F.);
#11863=ORIENTED_EDGE('',*,*,#7968,.F.);
#11864=ORIENTED_EDGE('',*,*,#7982,.T.);
#11865=ORIENTED_EDGE('',*,*,#7895,.F.);
#11866=ORIENTED_EDGE('',*,*,#7983,.F.);
#11867=ORIENTED_EDGE('',*,*,#7961,.F.);
#11868=ORIENTED_EDGE('',*,*,#7984,.F.);
#11869=ORIENTED_EDGE('',*,*,#7897,.F.);
#11870=ORIENTED_EDGE('',*,*,#7985,.T.);
#11871=ORIENTED_EDGE('',*,*,#7959,.F.);
#11872=ORIENTED_EDGE('',*,*,#7958,.T.);
#11873=ORIENTED_EDGE('',*,*,#7983,.T.);
#11874=ORIENTED_EDGE('',*,*,#7894,.T.);
#11875=ORIENTED_EDGE('',*,*,#7984,.T.);
#11876=ORIENTED_EDGE('',*,*,#7985,.F.);
#11877=ORIENTED_EDGE('',*,*,#7896,.F.);
#11878=ORIENTED_EDGE('',*,*,#7982,.F.);
#11879=ORIENTED_EDGE('',*,*,#7960,.F.);
#11880=ORIENTED_EDGE('',*,*,#7986,.T.);
#11881=ORIENTED_EDGE('',*,*,#7907,.F.);
#11882=ORIENTED_EDGE('',*,*,#7987,.F.);
#11883=ORIENTED_EDGE('',*,*,#7973,.F.);
#11884=ORIENTED_EDGE('',*,*,#7988,.F.);
#11885=ORIENTED_EDGE('',*,*,#7909,.F.);
#11886=ORIENTED_EDGE('',*,*,#7989,.T.);
#11887=ORIENTED_EDGE('',*,*,#7971,.F.);
#11888=ORIENTED_EDGE('',*,*,#7970,.T.);
#11889=ORIENTED_EDGE('',*,*,#7987,.T.);
#11890=ORIENTED_EDGE('',*,*,#7906,.T.);
#11891=ORIENTED_EDGE('',*,*,#7988,.T.);
#11892=ORIENTED_EDGE('',*,*,#7989,.F.);
#11893=ORIENTED_EDGE('',*,*,#7908,.F.);
#11894=ORIENTED_EDGE('',*,*,#7986,.F.);
#11895=ORIENTED_EDGE('',*,*,#7972,.F.);
#11896=ORIENTED_EDGE('',*,*,#7990,.T.);
#11897=ORIENTED_EDGE('',*,*,#7889,.F.);
#11898=ORIENTED_EDGE('',*,*,#7991,.F.);
#11899=ORIENTED_EDGE('',*,*,#7935,.F.);
#11900=ORIENTED_EDGE('',*,*,#7992,.F.);
#11901=ORIENTED_EDGE('',*,*,#7887,.F.);
#11902=ORIENTED_EDGE('',*,*,#7993,.T.);
#11903=ORIENTED_EDGE('',*,*,#7937,.F.);
#11904=ORIENTED_EDGE('',*,*,#7936,.T.);
#11905=ORIENTED_EDGE('',*,*,#7991,.T.);
#11906=ORIENTED_EDGE('',*,*,#7888,.T.);
#11907=ORIENTED_EDGE('',*,*,#7992,.T.);
#11908=ORIENTED_EDGE('',*,*,#7993,.F.);
#11909=ORIENTED_EDGE('',*,*,#7886,.F.);
#11910=ORIENTED_EDGE('',*,*,#7990,.F.);
#11911=ORIENTED_EDGE('',*,*,#7934,.F.);
#11912=ORIENTED_EDGE('',*,*,#7994,.T.);
#11913=ORIENTED_EDGE('',*,*,#7919,.F.);
#11914=ORIENTED_EDGE('',*,*,#7995,.F.);
#11915=ORIENTED_EDGE('',*,*,#7949,.F.);
#11916=ORIENTED_EDGE('',*,*,#7996,.F.);
#11917=ORIENTED_EDGE('',*,*,#7921,.F.);
#11918=ORIENTED_EDGE('',*,*,#7997,.T.);
#11919=ORIENTED_EDGE('',*,*,#7947,.F.);
#11920=ORIENTED_EDGE('',*,*,#7946,.T.);
#11921=ORIENTED_EDGE('',*,*,#7995,.T.);
#11922=ORIENTED_EDGE('',*,*,#7918,.T.);
#11923=ORIENTED_EDGE('',*,*,#7996,.T.);
#11924=ORIENTED_EDGE('',*,*,#7997,.F.);
#11925=ORIENTED_EDGE('',*,*,#7920,.F.);
#11926=ORIENTED_EDGE('',*,*,#7994,.F.);
#11927=ORIENTED_EDGE('',*,*,#7948,.F.);
#11928=ORIENTED_EDGE('',*,*,#7998,.T.);
#11929=ORIENTED_EDGE('',*,*,#7915,.F.);
#11930=ORIENTED_EDGE('',*,*,#7999,.F.);
#11931=ORIENTED_EDGE('',*,*,#7945,.F.);
#11932=ORIENTED_EDGE('',*,*,#8000,.F.);
#11933=ORIENTED_EDGE('',*,*,#7917,.F.);
#11934=ORIENTED_EDGE('',*,*,#8001,.T.);
#11935=ORIENTED_EDGE('',*,*,#7943,.F.);
#11936=ORIENTED_EDGE('',*,*,#7942,.T.);
#11937=ORIENTED_EDGE('',*,*,#7999,.T.);
#11938=ORIENTED_EDGE('',*,*,#7914,.T.);
#11939=ORIENTED_EDGE('',*,*,#8000,.T.);
#11940=ORIENTED_EDGE('',*,*,#8001,.F.);
#11941=ORIENTED_EDGE('',*,*,#7916,.F.);
#11942=ORIENTED_EDGE('',*,*,#7998,.F.);
#11943=ORIENTED_EDGE('',*,*,#7944,.F.);
#11944=ORIENTED_EDGE('',*,*,#8002,.T.);
#11945=ORIENTED_EDGE('',*,*,#7923,.F.);
#11946=ORIENTED_EDGE('',*,*,#8003,.F.);
#11947=ORIENTED_EDGE('',*,*,#7953,.F.);
#11948=ORIENTED_EDGE('',*,*,#8004,.F.);
#11949=ORIENTED_EDGE('',*,*,#7925,.F.);
#11950=ORIENTED_EDGE('',*,*,#8005,.T.);
#11951=ORIENTED_EDGE('',*,*,#7951,.F.);
#11952=ORIENTED_EDGE('',*,*,#7950,.T.);
#11953=ORIENTED_EDGE('',*,*,#8003,.T.);
#11954=ORIENTED_EDGE('',*,*,#7922,.T.);
#11955=ORIENTED_EDGE('',*,*,#8004,.T.);
#11956=ORIENTED_EDGE('',*,*,#8005,.F.);
#11957=ORIENTED_EDGE('',*,*,#7924,.F.);
#11958=ORIENTED_EDGE('',*,*,#8002,.F.);
#11959=ORIENTED_EDGE('',*,*,#7952,.F.);
#11960=ORIENTED_EDGE('',*,*,#8006,.T.);
#11961=ORIENTED_EDGE('',*,*,#7911,.F.);
#11962=ORIENTED_EDGE('',*,*,#8007,.F.);
#11963=ORIENTED_EDGE('',*,*,#7941,.F.);
#11964=ORIENTED_EDGE('',*,*,#8008,.F.);
#11965=ORIENTED_EDGE('',*,*,#7913,.F.);
#11966=ORIENTED_EDGE('',*,*,#8009,.T.);
#11967=ORIENTED_EDGE('',*,*,#7939,.F.);
#11968=ORIENTED_EDGE('',*,*,#7938,.T.);
#11969=ORIENTED_EDGE('',*,*,#8007,.T.);
#11970=ORIENTED_EDGE('',*,*,#7910,.T.);
#11971=ORIENTED_EDGE('',*,*,#8008,.T.);
#11972=ORIENTED_EDGE('',*,*,#8009,.F.);
#11973=ORIENTED_EDGE('',*,*,#7912,.F.);
#11974=ORIENTED_EDGE('',*,*,#8006,.F.);
#11975=ORIENTED_EDGE('',*,*,#7940,.F.);
#11976=ORIENTED_EDGE('',*,*,#8010,.T.);
#11977=ORIENTED_EDGE('',*,*,#7884,.F.);
#11978=ORIENTED_EDGE('',*,*,#8011,.F.);
#11979=ORIENTED_EDGE('',*,*,#7932,.F.);
#11980=ORIENTED_EDGE('',*,*,#8012,.F.);
#11981=ORIENTED_EDGE('',*,*,#7880,.F.);
#11982=ORIENTED_EDGE('',*,*,#8013,.T.);
#11983=ORIENTED_EDGE('',*,*,#7928,.F.);
#11984=ORIENTED_EDGE('',*,*,#7927,.T.);
#11985=ORIENTED_EDGE('',*,*,#7933,.T.);
#11986=ORIENTED_EDGE('',*,*,#8011,.T.);
#11987=ORIENTED_EDGE('',*,*,#7883,.T.);
#11988=ORIENTED_EDGE('',*,*,#7881,.T.);
#11989=ORIENTED_EDGE('',*,*,#8012,.T.);
#11990=ORIENTED_EDGE('',*,*,#8013,.F.);
#11991=ORIENTED_EDGE('',*,*,#7879,.F.);
#11992=ORIENTED_EDGE('',*,*,#7885,.F.);
#11993=ORIENTED_EDGE('',*,*,#8010,.F.);
#11994=ORIENTED_EDGE('',*,*,#7931,.F.);
#11995=ORIENTED_EDGE('',*,*,#7929,.F.);
#11996=ORIENTED_EDGE('',*,*,#8014,.T.);
#11997=ORIENTED_EDGE('',*,*,#7891,.F.);
#11998=ORIENTED_EDGE('',*,*,#8015,.F.);
#11999=ORIENTED_EDGE('',*,*,#7957,.F.);
#12000=ORIENTED_EDGE('',*,*,#8016,.F.);
#12001=ORIENTED_EDGE('',*,*,#7893,.F.);
#12002=ORIENTED_EDGE('',*,*,#8017,.T.);
#12003=ORIENTED_EDGE('',*,*,#7955,.F.);
#12004=ORIENTED_EDGE('',*,*,#7954,.T.);
#12005=ORIENTED_EDGE('',*,*,#8015,.T.);
#12006=ORIENTED_EDGE('',*,*,#7890,.T.);
#12007=ORIENTED_EDGE('',*,*,#8016,.T.);
#12008=ORIENTED_EDGE('',*,*,#8017,.F.);
#12009=ORIENTED_EDGE('',*,*,#7892,.F.);
#12010=ORIENTED_EDGE('',*,*,#8014,.F.);
#12011=ORIENTED_EDGE('',*,*,#7956,.F.);
#12012=ORIENTED_EDGE('',*,*,#8018,.F.);
#12013=ORIENTED_EDGE('',*,*,#8019,.T.);
#12014=ORIENTED_EDGE('',*,*,#8020,.F.);
#12015=ORIENTED_EDGE('',*,*,#8021,.F.);
#12016=ORIENTED_EDGE('',*,*,#8019,.F.);
#12017=ORIENTED_EDGE('',*,*,#8022,.F.);
#12018=ORIENTED_EDGE('',*,*,#8023,.T.);
#12019=ORIENTED_EDGE('',*,*,#8024,.F.);
#12020=ORIENTED_EDGE('',*,*,#8023,.F.);
#12021=ORIENTED_EDGE('',*,*,#8025,.F.);
#12022=ORIENTED_EDGE('',*,*,#8026,.T.);
#12023=ORIENTED_EDGE('',*,*,#8027,.T.);
#12024=ORIENTED_EDGE('',*,*,#8028,.T.);
#12025=ORIENTED_EDGE('',*,*,#8026,.F.);
#12026=ORIENTED_EDGE('',*,*,#8029,.T.);
#12027=ORIENTED_EDGE('',*,*,#8030,.T.);
#12028=ORIENTED_EDGE('',*,*,#8027,.F.);
#12029=ORIENTED_EDGE('',*,*,#8028,.F.);
#12030=ORIENTED_EDGE('',*,*,#8030,.F.);
#12031=ORIENTED_EDGE('',*,*,#8031,.T.);
#12032=ORIENTED_EDGE('',*,*,#8029,.F.);
#12033=ORIENTED_EDGE('',*,*,#8032,.T.);
#12034=ORIENTED_EDGE('',*,*,#8033,.T.);
#12035=ORIENTED_EDGE('',*,*,#8032,.F.);
#12036=ORIENTED_EDGE('',*,*,#8031,.F.);
#12037=ORIENTED_EDGE('',*,*,#8033,.F.);
#12038=ORIENTED_EDGE('',*,*,#8034,.T.);
#12039=ORIENTED_EDGE('',*,*,#8035,.T.);
#12040=ORIENTED_EDGE('',*,*,#8034,.F.);
#12041=ORIENTED_EDGE('',*,*,#8024,.T.);
#12042=ORIENTED_EDGE('',*,*,#8036,.T.);
#12043=ORIENTED_EDGE('',*,*,#8020,.T.);
#12044=ORIENTED_EDGE('',*,*,#8021,.T.);
#12045=ORIENTED_EDGE('',*,*,#8036,.F.);
#12046=ORIENTED_EDGE('',*,*,#8037,.F.);
#12047=ORIENTED_EDGE('',*,*,#8038,.T.);
#12048=ORIENTED_EDGE('',*,*,#8025,.T.);
#12049=ORIENTED_EDGE('',*,*,#8038,.F.);
#12050=ORIENTED_EDGE('',*,*,#8037,.T.);
#12051=ORIENTED_EDGE('',*,*,#8018,.T.);
#12052=ORIENTED_EDGE('',*,*,#8035,.F.);
#12053=ORIENTED_EDGE('',*,*,#8022,.T.);
#12054=ORIENTED_EDGE('',*,*,#8039,.F.);
#12055=ORIENTED_EDGE('',*,*,#8040,.T.);
#12056=ORIENTED_EDGE('',*,*,#8041,.T.);
#12057=ORIENTED_EDGE('',*,*,#8040,.F.);
#12058=ORIENTED_EDGE('',*,*,#8041,.F.);
#12059=ORIENTED_EDGE('',*,*,#8039,.T.);
#12060=ORIENTED_EDGE('',*,*,#8042,.F.);
#12061=ORIENTED_EDGE('',*,*,#8043,.T.);
#12062=ORIENTED_EDGE('',*,*,#8044,.T.);
#12063=ORIENTED_EDGE('',*,*,#8043,.F.);
#12064=ORIENTED_EDGE('',*,*,#8044,.F.);
#12065=ORIENTED_EDGE('',*,*,#8042,.T.);
#12066=ORIENTED_EDGE('',*,*,#8045,.F.);
#12067=ORIENTED_EDGE('',*,*,#8046,.T.);
#12068=ORIENTED_EDGE('',*,*,#8047,.T.);
#12069=ORIENTED_EDGE('',*,*,#8046,.F.);
#12070=ORIENTED_EDGE('',*,*,#8047,.F.);
#12071=ORIENTED_EDGE('',*,*,#8045,.T.);
#12072=ORIENTED_EDGE('',*,*,#8048,.F.);
#12073=ORIENTED_EDGE('',*,*,#8049,.T.);
#12074=ORIENTED_EDGE('',*,*,#8050,.T.);
#12075=ORIENTED_EDGE('',*,*,#8049,.F.);
#12076=ORIENTED_EDGE('',*,*,#8050,.F.);
#12077=ORIENTED_EDGE('',*,*,#8048,.T.);
#12078=ORIENTED_EDGE('',*,*,#8051,.F.);
#12079=ORIENTED_EDGE('',*,*,#8052,.T.);
#12080=ORIENTED_EDGE('',*,*,#8053,.T.);
#12081=ORIENTED_EDGE('',*,*,#8052,.F.);
#12082=ORIENTED_EDGE('',*,*,#8053,.F.);
#12083=ORIENTED_EDGE('',*,*,#8051,.T.);
#12084=ORIENTED_EDGE('',*,*,#8054,.F.);
#12085=ORIENTED_EDGE('',*,*,#8055,.T.);
#12086=ORIENTED_EDGE('',*,*,#8056,.T.);
#12087=ORIENTED_EDGE('',*,*,#8055,.F.);
#12088=ORIENTED_EDGE('',*,*,#8056,.F.);
#12089=ORIENTED_EDGE('',*,*,#8054,.T.);
#12090=ORIENTED_EDGE('',*,*,#8057,.F.);
#12091=ORIENTED_EDGE('',*,*,#8058,.T.);
#12092=ORIENTED_EDGE('',*,*,#8059,.T.);
#12093=ORIENTED_EDGE('',*,*,#8058,.F.);
#12094=ORIENTED_EDGE('',*,*,#8059,.F.);
#12095=ORIENTED_EDGE('',*,*,#8057,.T.);
#12096=ORIENTED_EDGE('',*,*,#8060,.F.);
#12097=ORIENTED_EDGE('',*,*,#8061,.T.);
#12098=ORIENTED_EDGE('',*,*,#8062,.T.);
#12099=ORIENTED_EDGE('',*,*,#8061,.F.);
#12100=ORIENTED_EDGE('',*,*,#8062,.F.);
#12101=ORIENTED_EDGE('',*,*,#8060,.T.);
#12102=ORIENTED_EDGE('',*,*,#8063,.F.);
#12103=ORIENTED_EDGE('',*,*,#8064,.T.);
#12104=ORIENTED_EDGE('',*,*,#8065,.T.);
#12105=ORIENTED_EDGE('',*,*,#8064,.F.);
#12106=ORIENTED_EDGE('',*,*,#8065,.F.);
#12107=ORIENTED_EDGE('',*,*,#8063,.T.);
#12108=ORIENTED_EDGE('',*,*,#8066,.F.);
#12109=ORIENTED_EDGE('',*,*,#8067,.T.);
#12110=ORIENTED_EDGE('',*,*,#8068,.T.);
#12111=ORIENTED_EDGE('',*,*,#8067,.F.);
#12112=ORIENTED_EDGE('',*,*,#8068,.F.);
#12113=ORIENTED_EDGE('',*,*,#8066,.T.);
#12114=ORIENTED_EDGE('',*,*,#8069,.F.);
#12115=ORIENTED_EDGE('',*,*,#8070,.T.);
#12116=ORIENTED_EDGE('',*,*,#8071,.T.);
#12117=ORIENTED_EDGE('',*,*,#8070,.F.);
#12118=ORIENTED_EDGE('',*,*,#8071,.F.);
#12119=ORIENTED_EDGE('',*,*,#8069,.T.);
#12289=CYLINDRICAL_SURFACE('',#14128,20.);
#12290=CYLINDRICAL_SURFACE('',#14200,2.74859462638384);
#12291=CYLINDRICAL_SURFACE('',#14203,2.74859462638384);
#12292=CYLINDRICAL_SURFACE('',#14208,2.74859462638384);
#12293=CYLINDRICAL_SURFACE('',#14211,2.74859462638384);
#12294=CYLINDRICAL_SURFACE('',#14216,2.74859462638384);
#12295=CYLINDRICAL_SURFACE('',#14219,2.74859462638384);
#12296=CYLINDRICAL_SURFACE('',#14224,2.74859462638384);
#12297=CYLINDRICAL_SURFACE('',#14227,2.74859462638384);
#12298=CYLINDRICAL_SURFACE('',#14232,2.74859462638384);
#12299=CYLINDRICAL_SURFACE('',#14235,2.74859462638384);
#12300=CYLINDRICAL_SURFACE('',#14240,2.74859462638384);
#12301=CYLINDRICAL_SURFACE('',#14243,2.74859462638384);
#12302=CYLINDRICAL_SURFACE('',#14248,2.74859462638384);
#12303=CYLINDRICAL_SURFACE('',#14251,2.74859462638384);
#12304=CYLINDRICAL_SURFACE('',#14256,2.74859462638384);
#12305=CYLINDRICAL_SURFACE('',#14259,2.74859462638384);
#12306=CYLINDRICAL_SURFACE('',#14264,2.74859462638384);
#12307=CYLINDRICAL_SURFACE('',#14267,2.74859462638384);
#12308=CYLINDRICAL_SURFACE('',#14272,2.74859462638384);
#12309=CYLINDRICAL_SURFACE('',#14275,2.74859462638384);
#12310=CYLINDRICAL_SURFACE('',#14280,2.74859462638384);
#12311=CYLINDRICAL_SURFACE('',#14283,2.74859462638384);
#12312=CYLINDRICAL_SURFACE('',#14306,14.0317131491268);
#12313=CYLINDRICAL_SURFACE('',#14308,8.5);
#12314=CYLINDRICAL_SURFACE('',#14309,11.9728634517814);
#12315=CYLINDRICAL_SURFACE('',#14313,2.62159462638384);
#12316=CYLINDRICAL_SURFACE('',#14318,2.62159462638384);
#12317=CYLINDRICAL_SURFACE('',#14323,2.62159462638384);
#12318=CYLINDRICAL_SURFACE('',#14328,2.62159462638384);
#12319=CYLINDRICAL_SURFACE('',#14333,2.62159462638384);
#12320=CYLINDRICAL_SURFACE('',#14338,2.62159462638384);
#12321=CYLINDRICAL_SURFACE('',#14343,2.62159462638384);
#12322=CYLINDRICAL_SURFACE('',#14348,2.62159462638384);
#12323=CYLINDRICAL_SURFACE('',#14353,2.62159462638384);
#12324=CYLINDRICAL_SURFACE('',#14358,2.62159462638384);
#12325=CYLINDRICAL_SURFACE('',#14363,2.62159462638384);
#12892=ADVANCED_FACE('',(#1362),#185,.T.);
#12893=ADVANCED_FACE('',(#1363),#186,.T.);
#12894=ADVANCED_FACE('',(#1364),#337,.F.);
#12895=ADVANCED_FACE('',(#1365),#12289,.T.);
#12896=ADVANCED_FACE('',(#1366,#416),#562,.F.);
#12897=ADVANCED_FACE('',(#1367,#417),#563,.F.);
#12898=ADVANCED_FACE('',(#1368),#338,.T.);
#12899=ADVANCED_FACE('',(#1369),#339,.T.);
#12900=ADVANCED_FACE('',(#1370),#187,.T.);
#12901=ADVANCED_FACE('',(#1371),#340,.F.);
#12902=ADVANCED_FACE('',(#1372),#341,.F.);
#12903=ADVANCED_FACE('',(#1373,#418,#419,#420,#421,#422,#423,#424,#425,
#426,#427),#342,.F.);
#12904=ADVANCED_FACE('',(#1374,#428,#429,#430,#431,#432,#433,#434,#435,
#436,#437),#343,.T.);
#12905=ADVANCED_FACE('',(#1375),#12290,.F.);
#12906=ADVANCED_FACE('',(#1376),#12291,.F.);
#12907=ADVANCED_FACE('',(#1377),#564,.T.);
#12908=ADVANCED_FACE('',(#1378),#565,.F.);
#12909=ADVANCED_FACE('',(#1379),#12292,.F.);
#12910=ADVANCED_FACE('',(#1380),#12293,.F.);
#12911=ADVANCED_FACE('',(#1381),#566,.T.);
#12912=ADVANCED_FACE('',(#1382),#567,.F.);
#12913=ADVANCED_FACE('',(#1383),#12294,.F.);
#12914=ADVANCED_FACE('',(#1384),#12295,.F.);
#12915=ADVANCED_FACE('',(#1385),#568,.T.);
#12916=ADVANCED_FACE('',(#1386),#569,.F.);
#12917=ADVANCED_FACE('',(#1387),#12296,.F.);
#12918=ADVANCED_FACE('',(#1388),#12297,.F.);
#12919=ADVANCED_FACE('',(#1389),#570,.T.);
#12920=ADVANCED_FACE('',(#1390),#571,.F.);
#12921=ADVANCED_FACE('',(#1391),#12298,.F.);
#12922=ADVANCED_FACE('',(#1392),#12299,.F.);
#12923=ADVANCED_FACE('',(#1393),#572,.T.);
#12924=ADVANCED_FACE('',(#1394),#573,.F.);
#12925=ADVANCED_FACE('',(#1395),#12300,.F.);
#12926=ADVANCED_FACE('',(#1396),#12301,.F.);
#12927=ADVANCED_FACE('',(#1397),#574,.T.);
#12928=ADVANCED_FACE('',(#1398),#575,.F.);
#12929=ADVANCED_FACE('',(#1399),#12302,.F.);
#12930=ADVANCED_FACE('',(#1400),#12303,.F.);
#12931=ADVANCED_FACE('',(#1401),#576,.T.);
#12932=ADVANCED_FACE('',(#1402),#577,.F.);
#12933=ADVANCED_FACE('',(#1403),#12304,.F.);
#12934=ADVANCED_FACE('',(#1404),#12305,.F.);
#12935=ADVANCED_FACE('',(#1405),#578,.T.);
#12936=ADVANCED_FACE('',(#1406),#579,.F.);
#12937=ADVANCED_FACE('',(#1407),#12306,.F.);
#12938=ADVANCED_FACE('',(#1408),#12307,.F.);
#12939=ADVANCED_FACE('',(#1409),#580,.T.);
#12940=ADVANCED_FACE('',(#1410),#581,.F.);
#12941=ADVANCED_FACE('',(#1411),#12308,.F.);
#12942=ADVANCED_FACE('',(#1412),#12309,.F.);
#12943=ADVANCED_FACE('',(#1413),#582,.T.);
#12944=ADVANCED_FACE('',(#1414),#583,.F.);
#12945=ADVANCED_FACE('',(#1415),#12310,.F.);
#12946=ADVANCED_FACE('',(#1416),#12311,.F.);
#12947=ADVANCED_FACE('',(#1417),#584,.T.);
#12948=ADVANCED_FACE('',(#1418),#585,.F.);
#12949=ADVANCED_FACE('',(#1419),#188,.T.);
#12950=ADVANCED_FACE('',(#1420),#189,.T.);
#12951=ADVANCED_FACE('',(#1421),#344,.T.);
#12952=ADVANCED_FACE('',(#1422),#345,.T.);
#12953=ADVANCED_FACE('',(#1423),#346,.F.);
#12954=ADVANCED_FACE('',(#1424),#12312,.T.);
#12955=ADVANCED_FACE('',(#1425),#12313,.F.);
#12956=ADVANCED_FACE('',(#1426),#12314,.T.);
#12957=ADVANCED_FACE('',(#1427,#438),#586,.F.);
#12958=ADVANCED_FACE('',(#1428,#439),#587,.F.);
#12959=ADVANCED_FACE('',(#1429),#12315,.T.);
#12960=ADVANCED_FACE('',(#1430),#588,.F.);
#12961=ADVANCED_FACE('',(#1431),#589,.T.);
#12962=ADVANCED_FACE('',(#1432),#12316,.T.);
#12963=ADVANCED_FACE('',(#1433),#590,.F.);
#12964=ADVANCED_FACE('',(#1434),#591,.T.);
#12965=ADVANCED_FACE('',(#1435),#12317,.T.);
#12966=ADVANCED_FACE('',(#1436),#592,.F.);
#12967=ADVANCED_FACE('',(#1437),#593,.T.);
#12968=ADVANCED_FACE('',(#1438),#12318,.T.);
#12969=ADVANCED_FACE('',(#1439),#594,.F.);
#12970=ADVANCED_FACE('',(#1440),#595,.T.);
#12971=ADVANCED_FACE('',(#1441),#12319,.T.);
#12972=ADVANCED_FACE('',(#1442),#596,.F.);
#12973=ADVANCED_FACE('',(#1443),#597,.T.);
#12974=ADVANCED_FACE('',(#1444),#12320,.T.);
#12975=ADVANCED_FACE('',(#1445),#598,.F.);
#12976=ADVANCED_FACE('',(#1446),#599,.T.);
#12977=ADVANCED_FACE('',(#1447),#12321,.T.);
#12978=ADVANCED_FACE('',(#1448),#600,.F.);
#12979=ADVANCED_FACE('',(#1449),#601,.T.);
#12980=ADVANCED_FACE('',(#1450),#12322,.T.);
#12981=ADVANCED_FACE('',(#1451),#602,.F.);
#12982=ADVANCED_FACE('',(#1452),#603,.T.);
#12983=ADVANCED_FACE('',(#1453),#12323,.T.);
#12984=ADVANCED_FACE('',(#1454),#604,.F.);
#12985=ADVANCED_FACE('',(#1455),#605,.T.);
#12986=ADVANCED_FACE('',(#1456),#12324,.T.);
#12987=ADVANCED_FACE('',(#1457),#606,.F.);
#12988=ADVANCED_FACE('',(#1458),#607,.T.);
#12989=ADVANCED_FACE('',(#1459),#12325,.T.);
#12990=ADVANCED_FACE('',(#1460),#608,.F.);
#12991=ADVANCED_FACE('',(#1461),#609,.T.);
#13013=CLOSED_SHELL('',(#12892,#12893,#12894,#12895,#12896,#12897));
#13014=CLOSED_SHELL('',(#12898,#12899,#12900,#12901,#12902,#12903,#12904,
#12905,#12906,#12907,#12908,#12909,#12910,#12911,#12912,#12913,#12914,#12915,
#12916,#12917,#12918,#12919,#12920,#12921,#12922,#12923,#12924,#12925,#12926,
#12927,#12928,#12929,#12930,#12931,#12932,#12933,#12934,#12935,#12936,#12937,
#12938,#12939,#12940,#12941,#12942,#12943,#12944,#12945,#12946,#12947,#12948));
#13015=CLOSED_SHELL('',(#12949,#12950,#12951,#12952,#12953,#12954,#12955,
#12956,#12957,#12958));
#13016=CLOSED_SHELL('',(#12959,#12960,#12961));
#13017=CLOSED_SHELL('',(#12962,#12963,#12964));
#13018=CLOSED_SHELL('',(#12965,#12966,#12967));
#13019=CLOSED_SHELL('',(#12968,#12969,#12970));
#13020=CLOSED_SHELL('',(#12971,#12972,#12973));
#13021=CLOSED_SHELL('',(#12974,#12975,#12976));
#13022=CLOSED_SHELL('',(#12977,#12978,#12979));
#13023=CLOSED_SHELL('',(#12980,#12981,#12982));
#13024=CLOSED_SHELL('',(#12983,#12984,#12985));
#13025=CLOSED_SHELL('',(#12986,#12987,#12988));
#13026=CLOSED_SHELL('',(#12989,#12990,#12991));
#14115=AXIS2_PLACEMENT_3D('',#87716,#16798,#16799);
#14116=AXIS2_PLACEMENT_3D('',#87717,#16800,#16801);
#14117=AXIS2_PLACEMENT_3D('',#87720,#16802,#16803);
#14118=AXIS2_PLACEMENT_3D('',#87721,#16804,#16805);
#14119=AXIS2_PLACEMENT_3D('',#87723,#16806,#16807);
#14120=AXIS2_PLACEMENT_3D('',#87724,#16808,#16809);
#14121=AXIS2_PLACEMENT_3D('',#87725,#16810,#16811);
#14122=AXIS2_PLACEMENT_3D('',#87727,#16812,#16813);
#14123=AXIS2_PLACEMENT_3D('',#87729,#16814,#16815);
#14124=AXIS2_PLACEMENT_3D('',#87730,#16816,#16817);
#14125=AXIS2_PLACEMENT_3D('',#87731,#16818,#16819);
#14126=AXIS2_PLACEMENT_3D('',#87733,#16820,#16821);
#14127=AXIS2_PLACEMENT_3D('',#87736,#16823,#16824);
#14128=AXIS2_PLACEMENT_3D('',#87737,#16825,#16826);
#14129=AXIS2_PLACEMENT_3D('',#87739,#16828,#16829);
#14130=AXIS2_PLACEMENT_3D('',#87740,#16830,#16831);
#14131=AXIS2_PLACEMENT_3D('',#87741,#16832,#16833);
#14132=AXIS2_PLACEMENT_3D('',#87744,#16834,#16835);
#14133=AXIS2_PLACEMENT_3D('',#87745,#16836,#16837);
#14134=AXIS2_PLACEMENT_3D('',#87749,#16839,#16840);
#14135=AXIS2_PLACEMENT_3D('',#87750,#16841,#16842);
#14136=AXIS2_PLACEMENT_3D('',#87751,#16843,#16844);
#14137=AXIS2_PLACEMENT_3D('',#87754,#16845,#16846);
#14138=AXIS2_PLACEMENT_3D('',#87755,#16847,#16848);
#14139=AXIS2_PLACEMENT_3D('',#87759,#16850,#16851);
#14140=AXIS2_PLACEMENT_3D('',#87760,#16852,#16853);
#14141=AXIS2_PLACEMENT_3D('',#87761,#16854,#16855);
#14142=AXIS2_PLACEMENT_3D('',#87763,#16856,#16857);
#14143=AXIS2_PLACEMENT_3D('',#87765,#16858,#16859);
#14144=AXIS2_PLACEMENT_3D('',#87767,#16860,#16861);
#14145=AXIS2_PLACEMENT_3D('',#87768,#16862,#16863);
#14146=AXIS2_PLACEMENT_3D('',#87769,#16864,#16865);
#14147=AXIS2_PLACEMENT_3D('',#87772,#16866,#16867);
#14148=AXIS2_PLACEMENT_3D('',#87773,#16868,#16869);
#14149=AXIS2_PLACEMENT_3D('',#87775,#16871,#16872);
#14150=AXIS2_PLACEMENT_3D('',#87777,#16874,#16875);
#14151=AXIS2_PLACEMENT_3D('',#87781,#16877,#16878);
#14152=AXIS2_PLACEMENT_3D('',#87791,#16879,#16880);
#14153=AXIS2_PLACEMENT_3D('',#87794,#16882,#16883);
#14154=AXIS2_PLACEMENT_3D('',#87803,#16884,#16885);
#14155=AXIS2_PLACEMENT_3D('',#87806,#16886,#16887);
#14156=AXIS2_PLACEMENT_3D('',#87816,#16888,#16889);
#14157=AXIS2_PLACEMENT_3D('',#87826,#16890,#16891);
#14158=AXIS2_PLACEMENT_3D('',#87836,#16892,#16893);
#14159=AXIS2_PLACEMENT_3D('',#87846,#16894,#16895);
#14160=AXIS2_PLACEMENT_3D('',#87856,#16896,#16897);
#14161=AXIS2_PLACEMENT_3D('',#87866,#16898,#16899);
#14162=AXIS2_PLACEMENT_3D('',#87876,#16900,#16901);
#14163=AXIS2_PLACEMENT_3D('',#87886,#16902,#16903);
#14164=AXIS2_PLACEMENT_3D('',#87896,#16904,#16905);
#14165=AXIS2_PLACEMENT_3D('',#87906,#16906,#16907);
#14166=AXIS2_PLACEMENT_3D('',#87916,#16908,#16909);
#14167=AXIS2_PLACEMENT_3D('',#87926,#16910,#16911);
#14168=AXIS2_PLACEMENT_3D('',#87936,#16912,#16913);
#14169=AXIS2_PLACEMENT_3D('',#87946,#16914,#16915);
#14170=AXIS2_PLACEMENT_3D('',#87956,#16916,#16917);
#14171=AXIS2_PLACEMENT_3D('',#87966,#16918,#16919);
#14172=AXIS2_PLACEMENT_3D('',#87976,#16920,#16921);
#14173=AXIS2_PLACEMENT_3D('',#87986,#16922,#16923);
#14174=AXIS2_PLACEMENT_3D('',#87996,#16924,#16925);
#14175=AXIS2_PLACEMENT_3D('',#88004,#16926,#16927);
#14176=AXIS2_PLACEMENT_3D('',#88008,#16929,#16930);
#14177=AXIS2_PLACEMENT_3D('',#88018,#16931,#16932);
#14178=AXIS2_PLACEMENT_3D('',#88021,#16934,#16935);
#14179=AXIS2_PLACEMENT_3D('',#88030,#16936,#16937);
#14180=AXIS2_PLACEMENT_3D('',#88033,#16938,#16939);
#14181=AXIS2_PLACEMENT_3D('',#88043,#16940,#16941);
#14182=AXIS2_PLACEMENT_3D('',#88053,#16942,#16943);
#14183=AXIS2_PLACEMENT_3D('',#88063,#16944,#16945);
#14184=AXIS2_PLACEMENT_3D('',#88073,#16946,#16947);
#14185=AXIS2_PLACEMENT_3D('',#88083,#16948,#16949);
#14186=AXIS2_PLACEMENT_3D('',#88093,#16950,#16951);
#14187=AXIS2_PLACEMENT_3D('',#88103,#16952,#16953);
#14188=AXIS2_PLACEMENT_3D('',#88113,#16954,#16955);
#14189=AXIS2_PLACEMENT_3D('',#88123,#16956,#16957);
#14190=AXIS2_PLACEMENT_3D('',#88133,#16958,#16959);
#14191=AXIS2_PLACEMENT_3D('',#88143,#16960,#16961);
#14192=AXIS2_PLACEMENT_3D('',#88153,#16962,#16963);
#14193=AXIS2_PLACEMENT_3D('',#88163,#16964,#16965);
#14194=AXIS2_PLACEMENT_3D('',#88173,#16966,#16967);
#14195=AXIS2_PLACEMENT_3D('',#88183,#16968,#16969);
#14196=AXIS2_PLACEMENT_3D('',#88193,#16970,#16971);
#14197=AXIS2_PLACEMENT_3D('',#88203,#16972,#16973);
#14198=AXIS2_PLACEMENT_3D('',#88213,#16974,#16975);
#14199=AXIS2_PLACEMENT_3D('',#88223,#16976,#16977);
#14200=AXIS2_PLACEMENT_3D('',#88231,#16978,#16979);
#14201=AXIS2_PLACEMENT_3D('',#88232,#16980,#16981);
#14202=AXIS2_PLACEMENT_3D('',#88233,#16982,#16983);
#14203=AXIS2_PLACEMENT_3D('',#88234,#16984,#16985);
#14204=AXIS2_PLACEMENT_3D('',#88235,#16986,#16987);
#14205=AXIS2_PLACEMENT_3D('',#88236,#16988,#16989);
#14206=AXIS2_PLACEMENT_3D('',#88237,#16990,#16991);
#14207=AXIS2_PLACEMENT_3D('',#88238,#16992,#16993);
#14208=AXIS2_PLACEMENT_3D('',#88239,#16994,#16995);
#14209=AXIS2_PLACEMENT_3D('',#88240,#16996,#16997);
#14210=AXIS2_PLACEMENT_3D('',#88241,#16998,#16999);
#14211=AXIS2_PLACEMENT_3D('',#88242,#17000,#17001);
#14212=AXIS2_PLACEMENT_3D('',#88243,#17002,#17003);
#14213=AXIS2_PLACEMENT_3D('',#88244,#17004,#17005);
#14214=AXIS2_PLACEMENT_3D('',#88245,#17006,#17007);
#14215=AXIS2_PLACEMENT_3D('',#88246,#17008,#17009);
#14216=AXIS2_PLACEMENT_3D('',#88247,#17010,#17011);
#14217=AXIS2_PLACEMENT_3D('',#88248,#17012,#17013);
#14218=AXIS2_PLACEMENT_3D('',#88249,#17014,#17015);
#14219=AXIS2_PLACEMENT_3D('',#88250,#17016,#17017);
#14220=AXIS2_PLACEMENT_3D('',#88251,#17018,#17019);
#14221=AXIS2_PLACEMENT_3D('',#88252,#17020,#17021);
#14222=AXIS2_PLACEMENT_3D('',#88253,#17022,#17023);
#14223=AXIS2_PLACEMENT_3D('',#88254,#17024,#17025);
#14224=AXIS2_PLACEMENT_3D('',#88255,#17026,#17027);
#14225=AXIS2_PLACEMENT_3D('',#88256,#17028,#17029);
#14226=AXIS2_PLACEMENT_3D('',#88257,#17030,#17031);
#14227=AXIS2_PLACEMENT_3D('',#88258,#17032,#17033);
#14228=AXIS2_PLACEMENT_3D('',#88259,#17034,#17035);
#14229=AXIS2_PLACEMENT_3D('',#88260,#17036,#17037);
#14230=AXIS2_PLACEMENT_3D('',#88261,#17038,#17039);
#14231=AXIS2_PLACEMENT_3D('',#88262,#17040,#17041);
#14232=AXIS2_PLACEMENT_3D('',#88263,#17042,#17043);
#14233=AXIS2_PLACEMENT_3D('',#88264,#17044,#17045);
#14234=AXIS2_PLACEMENT_3D('',#88265,#17046,#17047);
#14235=AXIS2_PLACEMENT_3D('',#88266,#17048,#17049);
#14236=AXIS2_PLACEMENT_3D('',#88267,#17050,#17051);
#14237=AXIS2_PLACEMENT_3D('',#88268,#17052,#17053);
#14238=AXIS2_PLACEMENT_3D('',#88269,#17054,#17055);
#14239=AXIS2_PLACEMENT_3D('',#88270,#17056,#17057);
#14240=AXIS2_PLACEMENT_3D('',#88271,#17058,#17059);
#14241=AXIS2_PLACEMENT_3D('',#88272,#17060,#17061);
#14242=AXIS2_PLACEMENT_3D('',#88273,#17062,#17063);
#14243=AXIS2_PLACEMENT_3D('',#88274,#17064,#17065);
#14244=AXIS2_PLACEMENT_3D('',#88275,#17066,#17067);
#14245=AXIS2_PLACEMENT_3D('',#88276,#17068,#17069);
#14246=AXIS2_PLACEMENT_3D('',#88277,#17070,#17071);
#14247=AXIS2_PLACEMENT_3D('',#88278,#17072,#17073);
#14248=AXIS2_PLACEMENT_3D('',#88279,#17074,#17075);
#14249=AXIS2_PLACEMENT_3D('',#88280,#17076,#17077);
#14250=AXIS2_PLACEMENT_3D('',#88281,#17078,#17079);
#14251=AXIS2_PLACEMENT_3D('',#88282,#17080,#17081);
#14252=AXIS2_PLACEMENT_3D('',#88283,#17082,#17083);
#14253=AXIS2_PLACEMENT_3D('',#88284,#17084,#17085);
#14254=AXIS2_PLACEMENT_3D('',#88285,#17086,#17087);
#14255=AXIS2_PLACEMENT_3D('',#88286,#17088,#17089);
#14256=AXIS2_PLACEMENT_3D('',#88287,#17090,#17091);
#14257=AXIS2_PLACEMENT_3D('',#88288,#17092,#17093);
#14258=AXIS2_PLACEMENT_3D('',#88289,#17094,#17095);
#14259=AXIS2_PLACEMENT_3D('',#88290,#17096,#17097);
#14260=AXIS2_PLACEMENT_3D('',#88291,#17098,#17099);
#14261=AXIS2_PLACEMENT_3D('',#88292,#17100,#17101);
#14262=AXIS2_PLACEMENT_3D('',#88293,#17102,#17103);
#14263=AXIS2_PLACEMENT_3D('',#88294,#17104,#17105);
#14264=AXIS2_PLACEMENT_3D('',#88295,#17106,#17107);
#14265=AXIS2_PLACEMENT_3D('',#88296,#17108,#17109);
#14266=AXIS2_PLACEMENT_3D('',#88297,#17110,#17111);
#14267=AXIS2_PLACEMENT_3D('',#88298,#17112,#17113);
#14268=AXIS2_PLACEMENT_3D('',#88299,#17114,#17115);
#14269=AXIS2_PLACEMENT_3D('',#88300,#17116,#17117);
#14270=AXIS2_PLACEMENT_3D('',#88301,#17118,#17119);
#14271=AXIS2_PLACEMENT_3D('',#88302,#17120,#17121);
#14272=AXIS2_PLACEMENT_3D('',#88303,#17122,#17123);
#14273=AXIS2_PLACEMENT_3D('',#88304,#17124,#17125);
#14274=AXIS2_PLACEMENT_3D('',#88305,#17126,#17127);
#14275=AXIS2_PLACEMENT_3D('',#88306,#17128,#17129);
#14276=AXIS2_PLACEMENT_3D('',#88307,#17130,#17131);
#14277=AXIS2_PLACEMENT_3D('',#88308,#17132,#17133);
#14278=AXIS2_PLACEMENT_3D('',#88309,#17134,#17135);
#14279=AXIS2_PLACEMENT_3D('',#88310,#17136,#17137);
#14280=AXIS2_PLACEMENT_3D('',#88311,#17138,#17139);
#14281=AXIS2_PLACEMENT_3D('',#88312,#17140,#17141);
#14282=AXIS2_PLACEMENT_3D('',#88313,#17142,#17143);
#14283=AXIS2_PLACEMENT_3D('',#88314,#17144,#17145);
#14284=AXIS2_PLACEMENT_3D('',#88315,#17146,#17147);
#14285=AXIS2_PLACEMENT_3D('',#88316,#17148,#17149);
#14286=AXIS2_PLACEMENT_3D('',#88317,#17150,#17151);
#14287=AXIS2_PLACEMENT_3D('',#88318,#17152,#17153);
#14288=AXIS2_PLACEMENT_3D('',#88319,#17154,#17155);
#14289=AXIS2_PLACEMENT_3D('',#88321,#17156,#17157);
#14290=AXIS2_PLACEMENT_3D('',#88323,#17158,#17159);
#14291=AXIS2_PLACEMENT_3D('',#88325,#17160,#17161);
#14292=AXIS2_PLACEMENT_3D('',#88326,#17162,#17163);
#14293=AXIS2_PLACEMENT_3D('',#88327,#17164,#17165);
#14294=AXIS2_PLACEMENT_3D('',#88329,#17166,#17167);
#14295=AXIS2_PLACEMENT_3D('',#88331,#17168,#17169);
#14296=AXIS2_PLACEMENT_3D('',#88332,#17170,#17171);
#14297=AXIS2_PLACEMENT_3D('',#88333,#17172,#17173);
#14298=AXIS2_PLACEMENT_3D('',#88335,#17174,#17175);
#14299=AXIS2_PLACEMENT_3D('',#88339,#17177,#17178);
#14300=AXIS2_PLACEMENT_3D('',#88340,#17179,#17180);
#14301=AXIS2_PLACEMENT_3D('',#88341,#17181,#17182);
#14302=AXIS2_PLACEMENT_3D('',#88344,#17183,#17184);
#14303=AXIS2_PLACEMENT_3D('',#88346,#17186,#17187);
#14304=AXIS2_PLACEMENT_3D('',#88347,#17188,#17189);
#14305=AXIS2_PLACEMENT_3D('',#88350,#17191,#17192);
#14306=AXIS2_PLACEMENT_3D('',#88351,#17193,#17194);
#14307=AXIS2_PLACEMENT_3D('',#88354,#17196,#17197);
#14308=AXIS2_PLACEMENT_3D('',#88355,#17198,#17199);
#14309=AXIS2_PLACEMENT_3D('',#88357,#17201,#17202);
#14310=AXIS2_PLACEMENT_3D('',#88359,#17203,#17204);
#14311=AXIS2_PLACEMENT_3D('',#88361,#17206,#17207);
#14312=AXIS2_PLACEMENT_3D('',#88362,#17208,#17209);
#14313=AXIS2_PLACEMENT_3D('',#88363,#17210,#17211);
#14314=AXIS2_PLACEMENT_3D('',#88365,#17212,#17213);
#14315=AXIS2_PLACEMENT_3D('',#88368,#17215,#17216);
#14316=AXIS2_PLACEMENT_3D('',#88369,#17217,#17218);
#14317=AXIS2_PLACEMENT_3D('',#88370,#17219,#17220);
#14318=AXIS2_PLACEMENT_3D('',#88371,#17221,#17222);
#14319=AXIS2_PLACEMENT_3D('',#88373,#17223,#17224);
#14320=AXIS2_PLACEMENT_3D('',#88376,#17226,#17227);
#14321=AXIS2_PLACEMENT_3D('',#88377,#17228,#17229);
#14322=AXIS2_PLACEMENT_3D('',#88378,#17230,#17231);
#14323=AXIS2_PLACEMENT_3D('',#88379,#17232,#17233);
#14324=AXIS2_PLACEMENT_3D('',#88381,#17234,#17235);
#14325=AXIS2_PLACEMENT_3D('',#88384,#17237,#17238);
#14326=AXIS2_PLACEMENT_3D('',#88385,#17239,#17240);
#14327=AXIS2_PLACEMENT_3D('',#88386,#17241,#17242);
#14328=AXIS2_PLACEMENT_3D('',#88387,#17243,#17244);
#14329=AXIS2_PLACEMENT_3D('',#88389,#17245,#17246);
#14330=AXIS2_PLACEMENT_3D('',#88392,#17248,#17249);
#14331=AXIS2_PLACEMENT_3D('',#88393,#17250,#17251);
#14332=AXIS2_PLACEMENT_3D('',#88394,#17252,#17253);
#14333=AXIS2_PLACEMENT_3D('',#88395,#17254,#17255);
#14334=AXIS2_PLACEMENT_3D('',#88397,#17256,#17257);
#14335=AXIS2_PLACEMENT_3D('',#88400,#17259,#17260);
#14336=AXIS2_PLACEMENT_3D('',#88401,#17261,#17262);
#14337=AXIS2_PLACEMENT_3D('',#88402,#17263,#17264);
#14338=AXIS2_PLACEMENT_3D('',#88403,#17265,#17266);
#14339=AXIS2_PLACEMENT_3D('',#88405,#17267,#17268);
#14340=AXIS2_PLACEMENT_3D('',#88408,#17270,#17271);
#14341=AXIS2_PLACEMENT_3D('',#88409,#17272,#17273);
#14342=AXIS2_PLACEMENT_3D('',#88410,#17274,#17275);
#14343=AXIS2_PLACEMENT_3D('',#88411,#17276,#17277);
#14344=AXIS2_PLACEMENT_3D('',#88413,#17278,#17279);
#14345=AXIS2_PLACEMENT_3D('',#88416,#17281,#17282);
#14346=AXIS2_PLACEMENT_3D('',#88417,#17283,#17284);
#14347=AXIS2_PLACEMENT_3D('',#88418,#17285,#17286);
#14348=AXIS2_PLACEMENT_3D('',#88419,#17287,#17288);
#14349=AXIS2_PLACEMENT_3D('',#88421,#17289,#17290);
#14350=AXIS2_PLACEMENT_3D('',#88424,#17292,#17293);
#14351=AXIS2_PLACEMENT_3D('',#88425,#17294,#17295);
#14352=AXIS2_PLACEMENT_3D('',#88426,#17296,#17297);
#14353=AXIS2_PLACEMENT_3D('',#88427,#17298,#17299);
#14354=AXIS2_PLACEMENT_3D('',#88429,#17300,#17301);
#14355=AXIS2_PLACEMENT_3D('',#88432,#17303,#17304);
#14356=AXIS2_PLACEMENT_3D('',#88433,#17305,#17306);
#14357=AXIS2_PLACEMENT_3D('',#88434,#17307,#17308);
#14358=AXIS2_PLACEMENT_3D('',#88435,#17309,#17310);
#14359=AXIS2_PLACEMENT_3D('',#88437,#17311,#17312);
#14360=AXIS2_PLACEMENT_3D('',#88440,#17314,#17315);
#14361=AXIS2_PLACEMENT_3D('',#88441,#17316,#17317);
#14362=AXIS2_PLACEMENT_3D('',#88442,#17318,#17319);
#14363=AXIS2_PLACEMENT_3D('',#88443,#17320,#17321);
#14364=AXIS2_PLACEMENT_3D('',#88445,#17322,#17323);
#14365=AXIS2_PLACEMENT_3D('',#88448,#17325,#17326);
#14366=AXIS2_PLACEMENT_3D('',#88449,#17327,#17328);
#14367=AXIS2_PLACEMENT_3D('',#88450,#17329,#17330);
#16798=DIRECTION('axis',(0.,0.,1.));
#16799=DIRECTION('refdir',(1.,0.,0.));
#16800=DIRECTION('center_axis',(0.,0.,-1.));
#16801=DIRECTION('ref_axis',(-1.,0.,0.));
#16802=DIRECTION('center_axis',(0.,0.,-1.));
#16803=DIRECTION('ref_axis',(-1.,0.,0.));
#16804=DIRECTION('center_axis',(0.,0.,-1.));
#16805=DIRECTION('ref_axis',(-1.,0.,0.));
#16806=DIRECTION('center_axis',(-1.22464679914735E-16,-1.,0.));
#16807=DIRECTION('ref_axis',(1.,-1.22464679914735E-16,0.));
#16808=DIRECTION('center_axis',(0.,0.,1.));
#16809=DIRECTION('ref_axis',(-1.,0.,0.));
#16810=DIRECTION('center_axis',(0.,0.,1.));
#16811=DIRECTION('ref_axis',(1.,0.,0.));
#16812=DIRECTION('center_axis',(0.,0.,1.));
#16813=DIRECTION('ref_axis',(1.,0.,0.));
#16814=DIRECTION('center_axis',(1.22464679914735E-16,-1.,0.));
#16815=DIRECTION('ref_axis',(-1.,-1.22464679914735E-16,0.));
#16816=DIRECTION('center_axis',(0.,0.,-1.));
#16817=DIRECTION('ref_axis',(1.,0.,0.));
#16818=DIRECTION('center_axis',(0.,0.,-1.));
#16819=DIRECTION('ref_axis',(-1.,0.,0.));
#16820=DIRECTION('center_axis',(0.,0.,1.));
#16821=DIRECTION('ref_axis',(1.,0.,0.));
#16822=DIRECTION('',(0.246660747381231,-3.02072294755719E-17,-0.96910189128973));
#16823=DIRECTION('center_axis',(0.,0.,1.));
#16824=DIRECTION('ref_axis',(1.,0.,0.));
#16825=DIRECTION('center_axis',(0.,0.,1.));
#16826=DIRECTION('ref_axis',(1.,0.,0.));
#16827=DIRECTION('',(0.,0.,-1.));
#16828=DIRECTION('center_axis',(0.,0.,-1.));
#16829=DIRECTION('ref_axis',(-1.,0.,0.));
#16830=DIRECTION('center_axis',(0.,0.,1.));
#16831=DIRECTION('ref_axis',(1.,0.,0.));
#16832=DIRECTION('center_axis',(0.,0.,1.));
#16833=DIRECTION('ref_axis',(1.,0.,0.));
#16834=DIRECTION('center_axis',(0.,0.,1.));
#16835=DIRECTION('ref_axis',(1.,0.,0.));
#16836=DIRECTION('center_axis',(0.,0.,1.));
#16837=DIRECTION('ref_axis',(1.,0.,0.));
#16838=DIRECTION('',(0.969101891289732,1.18680752921562E-16,-0.246660747381225));
#16839=DIRECTION('center_axis',(0.,0.,1.));
#16840=DIRECTION('ref_axis',(1.,0.,0.));
#16841=DIRECTION('center_axis',(0.,0.,1.));
#16842=DIRECTION('ref_axis',(1.,0.,0.));
#16843=DIRECTION('center_axis',(0.,0.,1.));
#16844=DIRECTION('ref_axis',(1.,0.,0.));
#16845=DIRECTION('center_axis',(0.,0.,1.));
#16846=DIRECTION('ref_axis',(1.,0.,0.));
#16847=DIRECTION('center_axis',(0.,0.,1.));
#16848=DIRECTION('ref_axis',(1.,0.,0.));
#16849=DIRECTION('',(0.96910189128973,1.18680752921561E-16,-0.246660747381235));
#16850=DIRECTION('center_axis',(0.,0.,1.));
#16851=DIRECTION('ref_axis',(1.,0.,0.));
#16852=DIRECTION('center_axis',(0.,0.,1.));
#16853=DIRECTION('ref_axis',(1.,0.,0.));
#16854=DIRECTION('center_axis',(0.,0.,1.));
#16855=DIRECTION('ref_axis',(1.,0.,0.));
#16856=DIRECTION('center_axis',(0.,0.,1.));
#16857=DIRECTION('ref_axis',(1.,0.,0.));
#16858=DIRECTION('center_axis',(1.22464679914735E-16,-1.,0.));
#16859=DIRECTION('ref_axis',(-1.,-1.22464679914735E-16,0.));
#16860=DIRECTION('center_axis',(0.,0.,1.));
#16861=DIRECTION('ref_axis',(1.,0.,0.));
#16862=DIRECTION('center_axis',(0.,0.,1.));
#16863=DIRECTION('ref_axis',(1.,0.,0.));
#16864=DIRECTION('center_axis',(0.,0.,1.));
#16865=DIRECTION('ref_axis',(1.,0.,0.));
#16866=DIRECTION('center_axis',(0.,0.,1.));
#16867=DIRECTION('ref_axis',(1.,0.,0.));
#16868=DIRECTION('center_axis',(0.,0.,1.));
#16869=DIRECTION('ref_axis',(1.,0.,0.));
#16870=DIRECTION('',(-0.969101891289729,-1.18680752921561E-16,0.246660747381235));
#16871=DIRECTION('center_axis',(0.,0.,-1.));
#16872=DIRECTION('ref_axis',(-1.,0.,0.));
#16873=DIRECTION('',(0.246660747381231,-3.02072294755719E-17,-0.96910189128973));
#16874=DIRECTION('center_axis',(0.,0.,-1.));
#16875=DIRECTION('ref_axis',(-1.,0.,0.));
#16876=DIRECTION('',(0.246660747381232,-3.0207229475572E-17,-0.96910189128973));
#16877=DIRECTION('center_axis',(0.24415009662832,-0.0351034843719286,-0.96910189128973));
#16878=DIRECTION('ref_axis',(0.959237831365939,-0.137917578929237,0.246660747381233));
#16879=DIRECTION('center_axis',(0.24415009662832,-0.0351034843719286,-0.96910189128973));
#16880=DIRECTION('ref_axis',(0.959237831365939,-0.137917578929239,0.246660747381233));
#16881=DIRECTION('',(0.246660747381232,-3.0207229475572E-17,-0.96910189128973));
#16882=DIRECTION('center_axis',(0.24415009662832,-0.0351034843719286,-0.96910189128973));
#16883=DIRECTION('ref_axis',(0.959237831365939,-0.137917578929239,0.246660747381233));
#16884=DIRECTION('center_axis',(0.24415009662832,-0.0351034843719286,-0.96910189128973));
#16885=DIRECTION('ref_axis',(0.959237831365939,-0.137917578929237,0.246660747381233));
#16886=DIRECTION('center_axis',(0.24415009662832,0.0351034843719251,0.96910189128973));
#16887=DIRECTION('ref_axis',(0.95923783136594,0.137917578929228,-0.246660747381232));
#16888=DIRECTION('center_axis',(0.24415009662832,0.0351034843719251,0.96910189128973));
#16889=DIRECTION('ref_axis',(0.95923783136594,0.137917578929228,-0.246660747381232));
#16890=DIRECTION('center_axis',(0.224370507816025,0.102466577580428,-0.969101891289731));
#16891=DIRECTION('ref_axis',(0.881526087075181,0.402579474771446,0.24666074738123));
#16892=DIRECTION('center_axis',(0.224370507816032,0.102466577580431,-0.969101891289729));
#16893=DIRECTION('ref_axis',(0.88152608707551,0.402579474770722,0.246660747381237));
#16894=DIRECTION('center_axis',(-0.224370507816021,0.10246657758043,-0.969101891289732));
#16895=DIRECTION('ref_axis',(0.881526087075442,-0.402579474770876,-0.246660747381227));
#16896=DIRECTION('center_axis',(-0.224370507816028,0.102466577580433,-0.96910189128973));
#16897=DIRECTION('ref_axis',(0.881526087075883,-0.402579474769905,-0.246660747381234));
#16898=DIRECTION('center_axis',(0.,0.246660747381227,-0.969101891289732));
#16899=DIRECTION('ref_axis',(8.8690509017592E-14,0.969101891289732,0.246660747381227));
#16900=DIRECTION('center_axis',(0.,0.24666074738123,-0.969101891289731));
#16901=DIRECTION('ref_axis',(3.83623821814746E-14,0.969101891289731,0.24666074738123));
#16902=DIRECTION('center_axis',(0.133354868098391,0.207504225145229,-0.969101891289734));
#16903=DIRECTION('ref_axis',(0.523936038703428,0.815260389721652,0.246660747381218));
#16904=DIRECTION('center_axis',(0.133354868098401,0.207504225145245,-0.969101891289729));
#16905=DIRECTION('ref_axis',(0.523936038704652,0.815260389720859,0.246660747381237));
#16906=DIRECTION('center_axis',(-0.133354868098395,0.207504225145243,-0.96910189128973));
#16907=DIRECTION('ref_axis',(-0.523936038705528,0.815260389720298,0.246660747381232));
#16908=DIRECTION('center_axis',(-0.133354868098395,0.207504225145243,-0.96910189128973));
#16909=DIRECTION('ref_axis',(-0.523936038704714,0.815260389720821,0.246660747381232));
#16910=DIRECTION('center_axis',(0.186413754843265,-0.161528438065564,-0.969101891289731));
#16911=DIRECTION('ref_axis',(0.732398341849721,-0.634626775795911,0.246660747381227));
#16912=DIRECTION('center_axis',(0.186413754843273,-0.161528438065571,-0.969101891289729));
#16913=DIRECTION('ref_axis',(0.73239834184858,-0.634626775797224,0.246660747381238));
#16914=DIRECTION('center_axis',(-0.0694923630321335,-0.236669253978789,
-0.969101891289731));
#16915=DIRECTION('ref_axis',(0.273027553673175,0.929846455408943,-0.246660747381229));
#16916=DIRECTION('center_axis',(-0.0694923630321349,-0.236669253978794,
-0.96910189128973));
#16917=DIRECTION('ref_axis',(0.273027553672585,0.929846455409115,-0.246660747381234));
#16918=DIRECTION('center_axis',(-0.186413754843274,-0.161528438065567,-0.969101891289729));
#16919=DIRECTION('ref_axis',(0.732398341847415,0.634626775798569,-0.246660747381236));
#16920=DIRECTION('center_axis',(-0.186413754843274,-0.161528438065567,-0.969101891289729));
#16921=DIRECTION('ref_axis',(0.732398341848765,0.634626775797011,-0.246660747381236));
#16922=DIRECTION('center_axis',(0.0694923630321279,-0.236669253978783,-0.969101891289733));
#16923=DIRECTION('ref_axis',(-0.273027553672171,0.92984645540924,-0.246660747381221));
#16924=DIRECTION('center_axis',(0.0694923630321317,-0.236669253978795,-0.96910189128973));
#16925=DIRECTION('ref_axis',(-0.273027553674098,0.929846455408671,-0.246660747381234));
#16926=DIRECTION('center_axis',(0.,0.,-1.));
#16927=DIRECTION('ref_axis',(-1.,0.,0.));
#16928=DIRECTION('',(-0.246660747381232,3.0207229475572E-17,0.96910189128973));
#16929=DIRECTION('center_axis',(-0.24415009662832,0.0351034843719286,0.96910189128973));
#16930=DIRECTION('ref_axis',(-0.959237831365939,0.137917578929236,-0.246660747381233));
#16931=DIRECTION('center_axis',(-0.24415009662832,0.0351034843719286,0.96910189128973));
#16932=DIRECTION('ref_axis',(0.959237831365939,-0.137917578929238,0.246660747381233));
#16933=DIRECTION('',(-0.246660747381232,3.0207229475572E-17,0.96910189128973));
#16934=DIRECTION('center_axis',(-0.24415009662832,0.0351034843719286,0.96910189128973));
#16935=DIRECTION('ref_axis',(0.959237831365939,-0.137917578929238,0.246660747381233));
#16936=DIRECTION('center_axis',(-0.24415009662832,0.0351034843719286,0.96910189128973));
#16937=DIRECTION('ref_axis',(-0.959237831365939,0.137917578929236,-0.246660747381233));
#16938=DIRECTION('center_axis',(-0.24415009662832,-0.0351034843719251,-0.96910189128973));
#16939=DIRECTION('ref_axis',(-0.959237831365942,-0.137917578929217,0.246660747381232));
#16940=DIRECTION('center_axis',(-0.24415009662832,-0.0351034843719251,-0.96910189128973));
#16941=DIRECTION('ref_axis',(-0.959237831365944,-0.137917578929203,0.246660747381232));
#16942=DIRECTION('center_axis',(-0.186413754843269,0.161528438065567,0.96910189128973));
#16943=DIRECTION('ref_axis',(0.732398341851905,-0.634626775793389,0.246660747381232));
#16944=DIRECTION('center_axis',(-0.18641375484327,0.161528438065568,0.96910189128973));
#16945=DIRECTION('ref_axis',(0.732398341848808,-0.634626775796962,0.246660747381234));
#16946=DIRECTION('center_axis',(0.0694923630321361,0.236669253978799,0.969101891289728));
#16947=DIRECTION('ref_axis',(-0.273027553673749,-0.929846455408772,0.246660747381239));
#16948=DIRECTION('center_axis',(0.0694923630321337,0.23666925397879,0.969101891289731));
#16949=DIRECTION('ref_axis',(-0.273027553671541,-0.929846455409422,0.24666074738123));
#16950=DIRECTION('center_axis',(0.186413754843279,0.161528438065572,0.969101891289727));
#16951=DIRECTION('ref_axis',(0.732398341849398,0.634626775796278,-0.246660747381243));
#16952=DIRECTION('center_axis',(0.186413754843268,0.161528438065562,0.969101891289731));
#16953=DIRECTION('ref_axis',(0.732398341848618,0.634626775797183,-0.246660747381228));
#16954=DIRECTION('center_axis',(-0.069492363032132,0.236669253978797,0.969101891289729));
#16955=DIRECTION('ref_axis',(0.273027553672181,-0.929846455409233,0.246660747381236));
#16956=DIRECTION('center_axis',(-0.0694923630321308,0.236669253978793,0.96910189128973));
#16957=DIRECTION('ref_axis',(0.273027553671897,-0.929846455409317,0.246660747381232));
#16958=DIRECTION('center_axis',(-0.224370507816038,-0.102466577580434,0.969101891289727));
#16959=DIRECTION('ref_axis',(0.881526087074927,0.402579474771994,0.246660747381244));
#16960=DIRECTION('center_axis',(-0.224370507816024,-0.102466577580427,0.969101891289731));
#16961=DIRECTION('ref_axis',(0.881526087075581,0.402579474770572,0.246660747381228));
#16962=DIRECTION('center_axis',(0.224370507816031,-0.102466577580435,0.969101891289729));
#16963=DIRECTION('ref_axis',(0.881526087074644,-0.402579474772618,-0.246660747381238));
#16964=DIRECTION('center_axis',(0.224370507816023,-0.102466577580431,0.969101891289731));
#16965=DIRECTION('ref_axis',(0.881526087074849,-0.402579474772174,-0.246660747381229));
#16966=DIRECTION('center_axis',(0.,-0.246660747381242,0.969101891289728));
#16967=DIRECTION('ref_axis',(-1.28897081029733E-13,-0.969101891289728,-0.246660747381242));
#16968=DIRECTION('center_axis',(0.,-0.246660747381226,0.969101891289732));
#16969=DIRECTION('ref_axis',(-1.10961688006709E-13,-0.969101891289732,-0.246660747381226));
#16970=DIRECTION('center_axis',(-0.133354868098397,-0.207504225145238,0.969101891289731));
#16971=DIRECTION('ref_axis',(-0.523936038702875,-0.815260389722004,-0.246660747381229));
#16972=DIRECTION('center_axis',(-0.133354868098399,-0.207504225145241,0.96910189128973));
#16973=DIRECTION('ref_axis',(-0.523936038705122,-0.815260389720558,-0.246660747381233));
#16974=DIRECTION('center_axis',(0.133354868098399,-0.207504225145248,0.969101891289729));
#16975=DIRECTION('ref_axis',(0.523936038703478,-0.815260389721613,-0.246660747381238));
#16976=DIRECTION('center_axis',(0.133354868098395,-0.207504225145243,0.96910189128973));
#16977=DIRECTION('ref_axis',(0.523936038706261,-0.815260389719827,-0.246660747381232));
#16978=DIRECTION('center_axis',(0.,-0.246660747381232,0.96910189128973));
#16979=DIRECTION('ref_axis',(0.,-0.96910189128973,-0.246660747381232));
#16980=DIRECTION('center_axis',(0.,-0.246660747381232,0.96910189128973));
#16981=DIRECTION('ref_axis',(0.,-0.96910189128973,-0.246660747381232));
#16982=DIRECTION('center_axis',(0.,-0.246660747381232,0.96910189128973));
#16983=DIRECTION('ref_axis',(0.,-0.96910189128973,-0.246660747381232));
#16984=DIRECTION('center_axis',(0.,-0.246660747381232,0.96910189128973));
#16985=DIRECTION('ref_axis',(0.,-0.96910189128973,-0.246660747381232));
#16986=DIRECTION('center_axis',(0.,-0.246660747381232,0.96910189128973));
#16987=DIRECTION('ref_axis',(0.,-0.96910189128973,-0.246660747381232));
#16988=DIRECTION('center_axis',(0.,-0.246660747381232,0.96910189128973));
#16989=DIRECTION('ref_axis',(0.,-0.96910189128973,-0.246660747381232));
#16990=DIRECTION('center_axis',(0.,-0.246660747381232,0.96910189128973));
#16991=DIRECTION('ref_axis',(0.,-0.96910189128973,-0.246660747381232));
#16992=DIRECTION('center_axis',(0.,-0.246660747381232,0.96910189128973));
#16993=DIRECTION('ref_axis',(0.,-0.96910189128973,-0.246660747381232));
#16994=DIRECTION('center_axis',(-0.133354868098398,-0.207504225145241,0.96910189128973));
#16995=DIRECTION('ref_axis',(6.64639222343535E-18,-0.977835574035122,-0.209374282449881));
#16996=DIRECTION('center_axis',(-0.133354868098398,-0.207504225145241,0.96910189128973));
#16997=DIRECTION('ref_axis',(-0.523936038704646,-0.815260389720864,-0.246660747381232));
#16998=DIRECTION('center_axis',(-0.133354868098398,-0.207504225145241,0.96910189128973));
#16999=DIRECTION('ref_axis',(-0.523936038704646,-0.815260389720864,-0.246660747381232));
#17000=DIRECTION('center_axis',(-0.133354868098398,-0.207504225145241,0.96910189128973));
#17001=DIRECTION('ref_axis',(6.64639222343535E-18,-0.977835574035122,-0.209374282449881));
#17002=DIRECTION('center_axis',(-0.133354868098398,-0.207504225145241,0.96910189128973));
#17003=DIRECTION('ref_axis',(-0.523936038704646,-0.815260389720864,-0.246660747381232));
#17004=DIRECTION('center_axis',(-0.133354868098398,-0.207504225145241,0.96910189128973));
#17005=DIRECTION('ref_axis',(-0.523936038704646,-0.815260389720864,-0.246660747381232));
#17006=DIRECTION('center_axis',(-0.133354868098398,-0.207504225145241,0.96910189128973));
#17007=DIRECTION('ref_axis',(-0.523936038704646,-0.815260389720864,-0.246660747381232));
#17008=DIRECTION('center_axis',(-0.133354868098398,-0.207504225145241,0.96910189128973));
#17009=DIRECTION('ref_axis',(-0.523936038704646,-0.815260389720864,-0.246660747381232));
#17010=DIRECTION('center_axis',(0.224370507816026,-0.102466577580432,0.96910189128973));
#17011=DIRECTION('ref_axis',(0.974229800751124,4.74361669806406E-17,-0.225557742780924));
#17012=DIRECTION('center_axis',(0.224370507816026,-0.102466577580432,0.96910189128973));
#17013=DIRECTION('ref_axis',(0.88152608707571,-0.402579474770286,-0.246660747381232));
#17014=DIRECTION('center_axis',(0.224370507816026,-0.102466577580432,0.96910189128973));
#17015=DIRECTION('ref_axis',(0.88152608707571,-0.402579474770287,-0.246660747381232));
#17016=DIRECTION('center_axis',(0.224370507816026,-0.102466577580432,0.96910189128973));
#17017=DIRECTION('ref_axis',(0.974229800751124,4.74361669806406E-17,-0.225557742780924));
#17018=DIRECTION('center_axis',(0.224370507816026,-0.102466577580432,0.96910189128973));
#17019=DIRECTION('ref_axis',(0.88152608707571,-0.402579474770287,-0.246660747381232));
#17020=DIRECTION('center_axis',(0.224370507816026,-0.102466577580432,0.96910189128973));
#17021=DIRECTION('ref_axis',(0.88152608707571,-0.402579474770286,-0.246660747381232));
#17022=DIRECTION('center_axis',(0.224370507816026,-0.102466577580432,0.96910189128973));
#17023=DIRECTION('ref_axis',(0.88152608707571,-0.402579474770286,-0.246660747381232));
#17024=DIRECTION('center_axis',(0.224370507816026,-0.102466577580432,0.96910189128973));
#17025=DIRECTION('ref_axis',(0.88152608707571,-0.402579474770286,-0.246660747381232));
#17026=DIRECTION('center_axis',(0.133354868098395,-0.207504225145243,0.96910189128973));
#17027=DIRECTION('ref_axis',(-9.26824837722223E-18,-0.977835574035122,-0.209374282449883));
#17028=DIRECTION('center_axis',(0.133354868098395,-0.207504225145243,0.96910189128973));
#17029=DIRECTION('ref_axis',(0.523936038704634,-0.815260389720872,-0.246660747381232));
#17030=DIRECTION('center_axis',(0.133354868098395,-0.207504225145243,0.96910189128973));
#17031=DIRECTION('ref_axis',(0.523936038704634,-0.815260389720872,-0.246660747381232));
#17032=DIRECTION('center_axis',(0.133354868098395,-0.207504225145243,0.96910189128973));
#17033=DIRECTION('ref_axis',(-9.26824837722223E-18,-0.977835574035122,-0.209374282449883));
#17034=DIRECTION('center_axis',(0.133354868098395,-0.207504225145243,0.96910189128973));
#17035=DIRECTION('ref_axis',(0.523936038704634,-0.815260389720872,-0.246660747381232));
#17036=DIRECTION('center_axis',(0.133354868098395,-0.207504225145243,0.96910189128973));
#17037=DIRECTION('ref_axis',(0.523936038704634,-0.815260389720872,-0.246660747381232));
#17038=DIRECTION('center_axis',(0.133354868098395,-0.207504225145243,0.96910189128973));
#17039=DIRECTION('ref_axis',(0.523936038704634,-0.815260389720872,-0.246660747381232));
#17040=DIRECTION('center_axis',(0.133354868098395,-0.207504225145243,0.96910189128973));
#17041=DIRECTION('ref_axis',(0.523936038704634,-0.815260389720872,-0.246660747381232));
#17042=DIRECTION('center_axis',(0.24415009662832,0.0351034843719251,0.96910189128973));
#17043=DIRECTION('ref_axis',(0.969699533821307,1.91055182786379E-17,-0.244300663336677));
#17044=DIRECTION('center_axis',(0.24415009662832,0.0351034843719251,0.96910189128973));
#17045=DIRECTION('ref_axis',(0.959237831365941,0.137917578929223,-0.246660747381232));
#17046=DIRECTION('center_axis',(0.24415009662832,0.0351034843719251,0.96910189128973));
#17047=DIRECTION('ref_axis',(0.959237831365941,0.137917578929223,-0.246660747381232));
#17048=DIRECTION('center_axis',(0.24415009662832,0.0351034843719251,0.96910189128973));
#17049=DIRECTION('ref_axis',(0.969699533821307,1.91055182786379E-17,-0.244300663336677));
#17050=DIRECTION('center_axis',(0.24415009662832,0.0351034843719251,0.96910189128973));
#17051=DIRECTION('ref_axis',(0.959237831365941,0.137917578929223,-0.246660747381232));
#17052=DIRECTION('center_axis',(0.24415009662832,0.0351034843719251,0.96910189128973));
#17053=DIRECTION('ref_axis',(0.959237831365941,0.137917578929223,-0.246660747381232));
#17054=DIRECTION('center_axis',(0.24415009662832,0.0351034843719251,0.96910189128973));
#17055=DIRECTION('ref_axis',(0.959237831365941,0.137917578929223,-0.246660747381232));
#17056=DIRECTION('center_axis',(0.24415009662832,0.0351034843719251,0.96910189128973));
#17057=DIRECTION('ref_axis',(0.959237831365941,0.137917578929223,-0.246660747381232));
#17058=DIRECTION('center_axis',(0.186413754843271,0.161528438065564,0.96910189128973));
#17059=DIRECTION('ref_axis',(0.981997424615724,-8.44807439072016E-17,-0.188894303905874));
#17060=DIRECTION('center_axis',(0.186413754843271,0.161528438065564,0.96910189128973));
#17061=DIRECTION('ref_axis',(0.732398341848126,0.63462677579775,-0.246660747381232));
#17062=DIRECTION('center_axis',(0.186413754843271,0.161528438065564,0.96910189128973));
#17063=DIRECTION('ref_axis',(0.732398341848126,0.63462677579775,-0.246660747381232));
#17064=DIRECTION('center_axis',(0.186413754843271,0.161528438065564,0.96910189128973));
#17065=DIRECTION('ref_axis',(0.981997424615724,-8.44807439072016E-17,-0.188894303905874));
#17066=DIRECTION('center_axis',(0.186413754843271,0.161528438065564,0.96910189128973));
#17067=DIRECTION('ref_axis',(0.732398341848126,0.63462677579775,-0.246660747381232));
#17068=DIRECTION('center_axis',(0.186413754843271,0.161528438065564,0.96910189128973));
#17069=DIRECTION('ref_axis',(0.732398341848126,0.63462677579775,-0.246660747381232));
#17070=DIRECTION('center_axis',(0.186413754843271,0.161528438065565,0.96910189128973));
#17071=DIRECTION('ref_axis',(0.732398341848126,0.63462677579775,-0.246660747381233));
#17072=DIRECTION('center_axis',(0.186413754843271,0.161528438065565,0.96910189128973));
#17073=DIRECTION('ref_axis',(0.732398341848126,0.63462677579775,-0.246660747381233));
#17074=DIRECTION('center_axis',(0.0694923630321343,0.236669253978792,0.96910189128973));
#17075=DIRECTION('ref_axis',(1.56176593776512E-18,-0.971450388587214,0.237242792332563));
#17076=DIRECTION('center_axis',(0.0694923630321343,0.236669253978792,0.96910189128973));
#17077=DIRECTION('ref_axis',(0.273027553672928,0.929846455409014,-0.246660747381232));
#17078=DIRECTION('center_axis',(0.0694923630321343,0.236669253978792,0.96910189128973));
#17079=DIRECTION('ref_axis',(0.273027553672928,0.929846455409015,-0.246660747381232));
#17080=DIRECTION('center_axis',(0.0694923630321343,0.236669253978792,0.96910189128973));
#17081=DIRECTION('ref_axis',(1.56176593776512E-18,-0.971450388587214,0.237242792332563));
#17082=DIRECTION('center_axis',(0.0694923630321343,0.236669253978792,0.96910189128973));
#17083=DIRECTION('ref_axis',(0.273027553672928,0.929846455409015,-0.246660747381232));
#17084=DIRECTION('center_axis',(0.0694923630321343,0.236669253978792,0.96910189128973));
#17085=DIRECTION('ref_axis',(0.273027553672928,0.929846455409014,-0.246660747381232));
#17086=DIRECTION('center_axis',(0.0694923630321343,0.236669253978792,0.96910189128973));
#17087=DIRECTION('ref_axis',(0.273027553672928,0.929846455409014,-0.246660747381232));
#17088=DIRECTION('center_axis',(0.0694923630321343,0.236669253978792,0.96910189128973));
#17089=DIRECTION('ref_axis',(0.273027553672928,0.929846455409014,-0.246660747381232));
#17090=DIRECTION('center_axis',(-0.0694923630321309,0.236669253978793,0.96910189128973));
#17091=DIRECTION('ref_axis',(4.13885935595183E-18,-0.971450388587214,0.237242792332564));
#17092=DIRECTION('center_axis',(-0.0694923630321309,0.236669253978793,0.96910189128973));
#17093=DIRECTION('ref_axis',(-0.273027553672915,0.929846455409018,-0.246660747381232));
#17094=DIRECTION('center_axis',(-0.0694923630321309,0.236669253978793,0.96910189128973));
#17095=DIRECTION('ref_axis',(-0.273027553672915,0.929846455409018,-0.246660747381232));
#17096=DIRECTION('center_axis',(-0.0694923630321309,0.236669253978793,0.96910189128973));
#17097=DIRECTION('ref_axis',(4.13885935595183E-18,-0.971450388587214,0.237242792332564));
#17098=DIRECTION('center_axis',(-0.0694923630321309,0.236669253978793,0.96910189128973));
#17099=DIRECTION('ref_axis',(-0.273027553672915,0.929846455409018,-0.246660747381232));
#17100=DIRECTION('center_axis',(-0.0694923630321309,0.236669253978793,0.96910189128973));
#17101=DIRECTION('ref_axis',(-0.273027553672915,0.929846455409018,-0.246660747381232));
#17102=DIRECTION('center_axis',(-0.0694923630321309,0.236669253978793,0.96910189128973));
#17103=DIRECTION('ref_axis',(-0.273027553672915,0.929846455409019,-0.246660747381232));
#17104=DIRECTION('center_axis',(-0.0694923630321309,0.236669253978793,0.96910189128973));
#17105=DIRECTION('ref_axis',(-0.273027553672915,0.929846455409019,-0.246660747381232));
#17106=DIRECTION('center_axis',(-0.186413754843268,0.161528438065567,0.96910189128973));
#17107=DIRECTION('ref_axis',(0.981997424615725,-7.60197659822491E-17,0.188894303905871));
#17108=DIRECTION('center_axis',(-0.186413754843269,0.161528438065567,0.96910189128973));
#17109=DIRECTION('ref_axis',(-0.732398341848117,0.63462677579776,-0.246660747381232));
#17110=DIRECTION('center_axis',(-0.186413754843269,0.161528438065567,0.96910189128973));
#17111=DIRECTION('ref_axis',(-0.732398341848117,0.63462677579776,-0.246660747381232));
#17112=DIRECTION('center_axis',(-0.186413754843268,0.161528438065567,0.96910189128973));
#17113=DIRECTION('ref_axis',(0.981997424615725,-7.60197659822491E-17,0.188894303905871));
#17114=DIRECTION('center_axis',(-0.186413754843269,0.161528438065567,0.96910189128973));
#17115=DIRECTION('ref_axis',(-0.732398341848117,0.63462677579776,-0.246660747381232));
#17116=DIRECTION('center_axis',(-0.186413754843269,0.161528438065567,0.96910189128973));
#17117=DIRECTION('ref_axis',(-0.732398341848117,0.63462677579776,-0.246660747381232));
#17118=DIRECTION('center_axis',(-0.186413754843269,0.161528438065567,0.96910189128973));
#17119=DIRECTION('ref_axis',(-0.732398341848117,0.63462677579776,-0.246660747381232));
#17120=DIRECTION('center_axis',(-0.186413754843269,0.161528438065567,0.96910189128973));
#17121=DIRECTION('ref_axis',(-0.732398341848117,0.63462677579776,-0.246660747381232));
#17122=DIRECTION('center_axis',(-0.24415009662832,0.0351034843719286,0.96910189128973));
#17123=DIRECTION('ref_axis',(0.969699533821307,2.42444443558668E-17,0.244300663336677));
#17124=DIRECTION('center_axis',(-0.24415009662832,0.0351034843719286,0.96910189128973));
#17125=DIRECTION('ref_axis',(-0.959237831365939,0.137917578929236,-0.246660747381233));
#17126=DIRECTION('center_axis',(-0.24415009662832,0.0351034843719286,0.96910189128973));
#17127=DIRECTION('ref_axis',(-0.959237831365939,0.137917578929236,-0.246660747381233));
#17128=DIRECTION('center_axis',(-0.24415009662832,0.0351034843719286,0.96910189128973));
#17129=DIRECTION('ref_axis',(0.969699533821307,2.42444443558668E-17,0.244300663336677));
#17130=DIRECTION('center_axis',(-0.24415009662832,0.0351034843719286,0.96910189128973));
#17131=DIRECTION('ref_axis',(-0.959237831365939,0.137917578929236,-0.246660747381233));
#17132=DIRECTION('center_axis',(-0.24415009662832,0.0351034843719286,0.96910189128973));
#17133=DIRECTION('ref_axis',(-0.959237831365939,0.137917578929236,-0.246660747381233));
#17134=DIRECTION('center_axis',(-0.24415009662832,0.0351034843719286,0.96910189128973));
#17135=DIRECTION('ref_axis',(-0.959237831365939,0.137917578929236,-0.246660747381233));
#17136=DIRECTION('center_axis',(-0.24415009662832,0.0351034843719286,0.96910189128973));
#17137=DIRECTION('ref_axis',(-0.959237831365939,0.137917578929236,-0.246660747381233));
#17138=DIRECTION('center_axis',(-0.224370507816027,-0.102466577580429,0.96910189128973));
#17139=DIRECTION('ref_axis',(0.974229800751124,3.55624843785764E-17,0.225557742780925));
#17140=DIRECTION('center_axis',(-0.224370507816027,-0.102466577580429,0.96910189128973));
#17141=DIRECTION('ref_axis',(-0.881526087075716,-0.402579474770274,-0.246660747381232));
#17142=DIRECTION('center_axis',(-0.224370507816027,-0.102466577580429,0.96910189128973));
#17143=DIRECTION('ref_axis',(-0.881526087075716,-0.402579474770274,-0.246660747381232));
#17144=DIRECTION('center_axis',(-0.224370507816027,-0.102466577580429,0.96910189128973));
#17145=DIRECTION('ref_axis',(0.974229800751124,3.55624843785764E-17,0.225557742780925));
#17146=DIRECTION('center_axis',(-0.224370507816027,-0.102466577580429,0.96910189128973));
#17147=DIRECTION('ref_axis',(-0.881526087075716,-0.402579474770274,-0.246660747381232));
#17148=DIRECTION('center_axis',(-0.224370507816027,-0.102466577580429,0.96910189128973));
#17149=DIRECTION('ref_axis',(-0.881526087075716,-0.402579474770274,-0.246660747381232));
#17150=DIRECTION('center_axis',(-0.224370507816027,-0.102466577580429,0.96910189128973));
#17151=DIRECTION('ref_axis',(-0.881526087075716,-0.402579474770274,-0.246660747381232));
#17152=DIRECTION('center_axis',(-0.224370507816027,-0.102466577580429,0.96910189128973));
#17153=DIRECTION('ref_axis',(-0.881526087075716,-0.402579474770274,-0.246660747381232));
#17154=DIRECTION('center_axis',(0.,0.,-1.));
#17155=DIRECTION('ref_axis',(-1.,0.,0.));
#17156=DIRECTION('center_axis',(0.,0.,-1.));
#17157=DIRECTION('ref_axis',(-1.,0.,0.));
#17158=DIRECTION('center_axis',(-1.22464679914735E-16,-1.,0.));
#17159=DIRECTION('ref_axis',(1.,-1.22464679914735E-16,0.));
#17160=DIRECTION('center_axis',(0.,0.,1.));
#17161=DIRECTION('ref_axis',(-1.,0.,0.));
#17162=DIRECTION('center_axis',(0.,0.,1.));
#17163=DIRECTION('ref_axis',(-1.,0.,0.));
#17164=DIRECTION('center_axis',(0.,0.,1.));
#17165=DIRECTION('ref_axis',(1.,0.,0.));
#17166=DIRECTION('center_axis',(0.,0.,1.));
#17167=DIRECTION('ref_axis',(1.,0.,0.));
#17168=DIRECTION('center_axis',(1.22464679914735E-16,-1.,0.));
#17169=DIRECTION('ref_axis',(-1.,-1.22464679914735E-16,0.));
#17170=DIRECTION('center_axis',(0.,0.,-1.));
#17171=DIRECTION('ref_axis',(1.,0.,0.));
#17172=DIRECTION('center_axis',(0.,0.,1.));
#17173=DIRECTION('ref_axis',(1.,0.,0.));
#17174=DIRECTION('center_axis',(0.,0.,1.));
#17175=DIRECTION('ref_axis',(1.,0.,0.));
#17176=DIRECTION('',(0.96910189128973,1.18680752921561E-16,-0.246660747381235));
#17177=DIRECTION('center_axis',(0.,0.,1.));
#17178=DIRECTION('ref_axis',(1.,0.,0.));
#17179=DIRECTION('center_axis',(0.,0.,1.));
#17180=DIRECTION('ref_axis',(1.,0.,0.));
#17181=DIRECTION('center_axis',(0.,0.,-1.));
#17182=DIRECTION('ref_axis',(-1.,0.,0.));
#17183=DIRECTION('center_axis',(0.,0.,1.));
#17184=DIRECTION('ref_axis',(1.,0.,0.));
#17185=DIRECTION('',(-0.246660747381233,3.02072294755721E-17,0.96910189128973));
#17186=DIRECTION('center_axis',(0.,0.,1.));
#17187=DIRECTION('ref_axis',(1.,0.,0.));
#17188=DIRECTION('center_axis',(0.,0.,1.));
#17189=DIRECTION('ref_axis',(1.,0.,0.));
#17190=DIRECTION('',(-0.96910189128973,-1.18680752921561E-16,0.246660747381235));
#17191=DIRECTION('center_axis',(0.,0.,1.));
#17192=DIRECTION('ref_axis',(1.,0.,0.));
#17193=DIRECTION('center_axis',(0.,0.,1.));
#17194=DIRECTION('ref_axis',(1.,0.,0.));
#17195=DIRECTION('',(0.,0.,-1.));
#17196=DIRECTION('center_axis',(0.,0.,1.));
#17197=DIRECTION('ref_axis',(1.,0.,0.));
#17198=DIRECTION('center_axis',(0.,0.,1.));
#17199=DIRECTION('ref_axis',(1.,0.,0.));
#17200=DIRECTION('',(0.,0.,1.));
#17201=DIRECTION('center_axis',(0.,0.,1.));
#17202=DIRECTION('ref_axis',(1.,0.,0.));
#17203=DIRECTION('center_axis',(0.,0.,1.));
#17204=DIRECTION('ref_axis',(1.,0.,0.));
#17205=DIRECTION('',(0.,0.,-1.));
#17206=DIRECTION('center_axis',(0.,0.,-1.));
#17207=DIRECTION('ref_axis',(-1.,0.,0.));
#17208=DIRECTION('center_axis',(0.,0.,1.));
#17209=DIRECTION('ref_axis',(1.,0.,0.));
#17210=DIRECTION('center_axis',(0.,-0.246660747381232,0.96910189128973));
#17211=DIRECTION('ref_axis',(0.,-0.96910189128973,-0.246660747381232));
#17212=DIRECTION('center_axis',(0.,-0.246660747381232,0.96910189128973));
#17213=DIRECTION('ref_axis',(0.,-0.96910189128973,-0.246660747381232));
#17214=DIRECTION('',(0.,0.246660747381232,-0.96910189128973));
#17215=DIRECTION('center_axis',(0.,-0.246660747381232,0.96910189128973));
#17216=DIRECTION('ref_axis',(0.,-0.96910189128973,-0.246660747381232));
#17217=DIRECTION('center_axis',(0.,-0.246660747381232,0.96910189128973));
#17218=DIRECTION('ref_axis',(0.,-0.96910189128973,-0.246660747381232));
#17219=DIRECTION('center_axis',(0.,-0.246660747381232,0.96910189128973));
#17220=DIRECTION('ref_axis',(0.,-0.96910189128973,-0.246660747381232));
#17221=DIRECTION('center_axis',(-0.133354868098398,-0.207504225145241,0.96910189128973));
#17222=DIRECTION('ref_axis',(-0.523936038704647,-0.815260389720864,-0.246660747381232));
#17223=DIRECTION('center_axis',(-0.133354868098398,-0.207504225145241,0.96910189128973));
#17224=DIRECTION('ref_axis',(-0.523936038704646,-0.815260389720864,-0.246660747381232));
#17225=DIRECTION('',(0.133354868098398,0.207504225145241,-0.96910189128973));
#17226=DIRECTION('center_axis',(-0.133354868098398,-0.207504225145241,0.96910189128973));
#17227=DIRECTION('ref_axis',(-0.523936038704646,-0.815260389720864,-0.246660747381232));
#17228=DIRECTION('center_axis',(-0.133354868098398,-0.207504225145241,0.96910189128973));
#17229=DIRECTION('ref_axis',(-0.523936038704646,-0.815260389720864,-0.246660747381232));
#17230=DIRECTION('center_axis',(-0.133354868098398,-0.207504225145241,0.96910189128973));
#17231=DIRECTION('ref_axis',(-0.523936038704646,-0.815260389720864,-0.246660747381232));
#17232=DIRECTION('center_axis',(-0.224370507816027,-0.102466577580429,0.96910189128973));
#17233=DIRECTION('ref_axis',(-0.881526087075716,-0.402579474770274,-0.246660747381232));
#17234=DIRECTION('center_axis',(-0.224370507816027,-0.102466577580429,0.96910189128973));
#17235=DIRECTION('ref_axis',(-0.881526087075716,-0.402579474770274,-0.246660747381232));
#17236=DIRECTION('',(0.224370507816027,0.102466577580429,-0.96910189128973));
#17237=DIRECTION('center_axis',(-0.224370507816027,-0.102466577580429,0.96910189128973));
#17238=DIRECTION('ref_axis',(-0.881526087075716,-0.402579474770274,-0.246660747381232));
#17239=DIRECTION('center_axis',(-0.224370507816027,-0.102466577580429,0.96910189128973));
#17240=DIRECTION('ref_axis',(-0.881526087075716,-0.402579474770274,-0.246660747381232));
#17241=DIRECTION('center_axis',(-0.224370507816027,-0.102466577580429,0.96910189128973));
#17242=DIRECTION('ref_axis',(-0.881526087075716,-0.402579474770274,-0.246660747381232));
#17243=DIRECTION('center_axis',(-0.244150096628319,0.0351034843719286,0.96910189128973));
#17244=DIRECTION('ref_axis',(-0.959237831365939,0.137917578929236,-0.246660747381232));
#17245=DIRECTION('center_axis',(-0.24415009662832,0.0351034843719286,0.96910189128973));
#17246=DIRECTION('ref_axis',(-0.959237831365939,0.137917578929236,-0.246660747381233));
#17247=DIRECTION('',(0.244150096628319,-0.0351034843719286,-0.96910189128973));
#17248=DIRECTION('center_axis',(-0.24415009662832,0.0351034843719286,0.96910189128973));
#17249=DIRECTION('ref_axis',(-0.959237831365939,0.137917578929236,-0.246660747381233));
#17250=DIRECTION('center_axis',(-0.24415009662832,0.0351034843719286,0.96910189128973));
#17251=DIRECTION('ref_axis',(-0.959237831365939,0.137917578929236,-0.246660747381233));
#17252=DIRECTION('center_axis',(-0.24415009662832,0.0351034843719286,0.96910189128973));
#17253=DIRECTION('ref_axis',(-0.959237831365939,0.137917578929236,-0.246660747381233));
#17254=DIRECTION('center_axis',(-0.186413754843269,0.161528438065567,0.96910189128973));
#17255=DIRECTION('ref_axis',(-0.732398341848117,0.63462677579776,-0.246660747381232));
#17256=DIRECTION('center_axis',(-0.186413754843269,0.161528438065567,0.96910189128973));
#17257=DIRECTION('ref_axis',(-0.732398341848117,0.63462677579776,-0.246660747381232));
#17258=DIRECTION('',(0.186413754843269,-0.161528438065567,-0.96910189128973));
#17259=DIRECTION('center_axis',(-0.186413754843269,0.161528438065567,0.96910189128973));
#17260=DIRECTION('ref_axis',(-0.732398341848117,0.634626775797761,-0.246660747381232));
#17261=DIRECTION('center_axis',(-0.186413754843269,0.161528438065567,0.96910189128973));
#17262=DIRECTION('ref_axis',(-0.732398341848117,0.63462677579776,-0.246660747381232));
#17263=DIRECTION('center_axis',(-0.186413754843269,0.161528438065567,0.96910189128973));
#17264=DIRECTION('ref_axis',(-0.732398341848117,0.63462677579776,-0.246660747381232));
#17265=DIRECTION('center_axis',(-0.0694923630321309,0.236669253978793,0.96910189128973));
#17266=DIRECTION('ref_axis',(-0.273027553672915,0.929846455409018,-0.246660747381232));
#17267=DIRECTION('center_axis',(-0.0694923630321309,0.236669253978793,0.96910189128973));
#17268=DIRECTION('ref_axis',(-0.273027553672915,0.929846455409018,-0.246660747381232));
#17269=DIRECTION('',(0.0694923630321309,-0.236669253978793,-0.96910189128973));
#17270=DIRECTION('center_axis',(-0.0694923630321309,0.236669253978793,0.96910189128973));
#17271=DIRECTION('ref_axis',(-0.273027553672915,0.929846455409018,-0.246660747381232));
#17272=DIRECTION('center_axis',(-0.0694923630321309,0.236669253978793,0.96910189128973));
#17273=DIRECTION('ref_axis',(-0.273027553672915,0.929846455409019,-0.246660747381232));
#17274=DIRECTION('center_axis',(-0.0694923630321309,0.236669253978793,0.96910189128973));
#17275=DIRECTION('ref_axis',(-0.273027553672915,0.929846455409019,-0.246660747381232));
#17276=DIRECTION('center_axis',(0.0694923630321343,0.236669253978792,0.96910189128973));
#17277=DIRECTION('ref_axis',(0.273027553672928,0.929846455409015,-0.246660747381232));
#17278=DIRECTION('center_axis',(0.0694923630321343,0.236669253978792,0.96910189128973));
#17279=DIRECTION('ref_axis',(0.273027553672928,0.929846455409015,-0.246660747381232));
#17280=DIRECTION('',(-0.0694923630321343,-0.236669253978792,-0.96910189128973));
#17281=DIRECTION('center_axis',(0.0694923630321343,0.236669253978792,0.96910189128973));
#17282=DIRECTION('ref_axis',(0.273027553672928,0.929846455409015,-0.246660747381232));
#17283=DIRECTION('center_axis',(0.0694923630321343,0.236669253978792,0.96910189128973));
#17284=DIRECTION('ref_axis',(0.273027553672928,0.929846455409014,-0.246660747381232));
#17285=DIRECTION('center_axis',(0.0694923630321343,0.236669253978792,0.96910189128973));
#17286=DIRECTION('ref_axis',(0.273027553672928,0.929846455409014,-0.246660747381232));
#17287=DIRECTION('center_axis',(0.186413754843271,0.161528438065564,0.96910189128973));
#17288=DIRECTION('ref_axis',(0.732398341848126,0.63462677579775,-0.246660747381232));
#17289=DIRECTION('center_axis',(0.186413754843271,0.161528438065564,0.96910189128973));
#17290=DIRECTION('ref_axis',(0.732398341848126,0.63462677579775,-0.246660747381232));
#17291=DIRECTION('',(-0.186413754843271,-0.161528438065564,-0.96910189128973));
#17292=DIRECTION('center_axis',(0.186413754843271,0.161528438065564,0.96910189128973));
#17293=DIRECTION('ref_axis',(0.732398341848126,0.63462677579775,-0.246660747381232));
#17294=DIRECTION('center_axis',(0.186413754843271,0.161528438065565,0.96910189128973));
#17295=DIRECTION('ref_axis',(0.732398341848126,0.63462677579775,-0.246660747381233));
#17296=DIRECTION('center_axis',(0.186413754843271,0.161528438065565,0.96910189128973));
#17297=DIRECTION('ref_axis',(0.732398341848126,0.63462677579775,-0.246660747381233));
#17298=DIRECTION('center_axis',(0.24415009662832,0.0351034843719251,0.96910189128973));
#17299=DIRECTION('ref_axis',(0.959237831365941,0.137917578929223,-0.246660747381232));
#17300=DIRECTION('center_axis',(0.24415009662832,0.0351034843719251,0.96910189128973));
#17301=DIRECTION('ref_axis',(0.959237831365941,0.137917578929223,-0.246660747381232));
#17302=DIRECTION('',(-0.24415009662832,-0.0351034843719251,-0.96910189128973));
#17303=DIRECTION('center_axis',(0.24415009662832,0.0351034843719251,0.96910189128973));
#17304=DIRECTION('ref_axis',(0.959237831365941,0.137917578929223,-0.246660747381232));
#17305=DIRECTION('center_axis',(0.24415009662832,0.0351034843719251,0.96910189128973));
#17306=DIRECTION('ref_axis',(0.959237831365941,0.137917578929223,-0.246660747381232));
#17307=DIRECTION('center_axis',(0.24415009662832,0.0351034843719251,0.96910189128973));
#17308=DIRECTION('ref_axis',(0.959237831365941,0.137917578929223,-0.246660747381232));
#17309=DIRECTION('center_axis',(0.224370507816026,-0.102466577580432,0.96910189128973));
#17310=DIRECTION('ref_axis',(0.88152608707571,-0.402579474770286,-0.246660747381232));
#17311=DIRECTION('center_axis',(0.224370507816026,-0.102466577580432,0.96910189128973));
#17312=DIRECTION('ref_axis',(0.88152608707571,-0.402579474770286,-0.246660747381232));
#17313=DIRECTION('',(-0.224370507816026,0.102466577580432,-0.96910189128973));
#17314=DIRECTION('center_axis',(0.224370507816026,-0.102466577580432,0.96910189128973));
#17315=DIRECTION('ref_axis',(0.88152608707571,-0.402579474770287,-0.246660747381232));
#17316=DIRECTION('center_axis',(0.224370507816026,-0.102466577580432,0.96910189128973));
#17317=DIRECTION('ref_axis',(0.88152608707571,-0.402579474770286,-0.246660747381232));
#17318=DIRECTION('center_axis',(0.224370507816026,-0.102466577580432,0.96910189128973));
#17319=DIRECTION('ref_axis',(0.88152608707571,-0.402579474770286,-0.246660747381232));
#17320=DIRECTION('center_axis',(0.133354868098395,-0.207504225145243,0.96910189128973));
#17321=DIRECTION('ref_axis',(0.523936038704634,-0.815260389720872,-0.246660747381232));
#17322=DIRECTION('center_axis',(0.133354868098395,-0.207504225145243,0.96910189128973));
#17323=DIRECTION('ref_axis',(0.523936038704634,-0.815260389720872,-0.246660747381232));
#17324=DIRECTION('',(-0.133354868098395,0.207504225145243,-0.96910189128973));
#17325=DIRECTION('center_axis',(0.133354868098395,-0.207504225145243,0.96910189128973));
#17326=DIRECTION('ref_axis',(0.523936038704634,-0.815260389720872,-0.246660747381232));
#17327=DIRECTION('center_axis',(0.133354868098395,-0.207504225145243,0.96910189128973));
#17328=DIRECTION('ref_axis',(0.523936038704634,-0.815260389720872,-0.246660747381232));
#17329=DIRECTION('center_axis',(0.133354868098395,-0.207504225145243,0.96910189128973));
#17330=DIRECTION('ref_axis',(0.523936038704634,-0.815260389720872,-0.246660747381232));
#87716=CARTESIAN_POINT('',(0.,0.,0.));
#87717=CARTESIAN_POINT('Origin',(0.,0.,5.225));
#87718=CARTESIAN_POINT('',(-20.,2.44929359829471E-15,5.225));
#87719=CARTESIAN_POINT('',(20.,-2.44929359829471E-15,5.225));
#87720=CARTESIAN_POINT('Origin',(0.,0.,5.225));
#87721=CARTESIAN_POINT('Origin',(0.,0.,5.225));
#87722=CARTESIAN_POINT('',(19.725,-2.41561581131815E-15,5.5));
#87723=CARTESIAN_POINT('Origin',(19.725,-2.41561581131815E-15,5.225));
#87724=CARTESIAN_POINT('Origin',(0.,0.,5.5));
#87725=CARTESIAN_POINT('Origin',(0.,0.,-5.225));
#87726=CARTESIAN_POINT('',(-20.,-2.44929359829471E-15,-5.225));
#87727=CARTESIAN_POINT('Origin',(0.,0.,-5.225));
#87728=CARTESIAN_POINT('',(-19.725,-2.41561581131815E-15,-5.5));
#87729=CARTESIAN_POINT('Origin',(-19.725,-2.41561581131815E-15,-5.225));
#87730=CARTESIAN_POINT('Origin',(0.,0.,-5.5));
#87731=CARTESIAN_POINT('Origin',(0.,0.,5.5));
#87732=CARTESIAN_POINT('',(15.4,-1.88595607068692E-15,5.5));
#87733=CARTESIAN_POINT('Origin',(0.,0.,5.5));
#87734=CARTESIAN_POINT('',(18.1997760045464,-2.22882974291666E-15,-5.5));
#87735=CARTESIAN_POINT('',(15.4,-1.88595607068692E-15,5.5));
#87736=CARTESIAN_POINT('Origin',(0.,0.,-5.5));
#87737=CARTESIAN_POINT('Origin',(0.,0.,4.25));
#87738=CARTESIAN_POINT('',(-20.,-2.44929359829471E-15,4.25));
#87739=CARTESIAN_POINT('Origin',(0.,15.4,5.5));
#87740=CARTESIAN_POINT('Origin',(0.,20.,-5.5));
#87741=CARTESIAN_POINT('Origin',(0.,0.,4.94191290631434));
#87742=CARTESIAN_POINT('',(13.0685506725942,1.81711532400453E-15,5.03423736132904));
#87743=CARTESIAN_POINT('',(-13.0685506725942,-1.60043587506875E-15,5.03423736132903));
#87744=CARTESIAN_POINT('Origin',(0.,0.,5.03423736132904));
#87745=CARTESIAN_POINT('Origin',(0.,0.,5.03423736132904));
#87746=CARTESIAN_POINT('',(-12.7058184384753,-1.55601398812262E-15,4.94191290631434));
#87747=CARTESIAN_POINT('',(-12.7058184384753,-1.55601398812262E-15,4.94191290631434));
#87748=CARTESIAN_POINT('',(12.7058184384753,1.55601398812262E-15,4.94191290631434));
#87749=CARTESIAN_POINT('Origin',(0.,0.,4.94191290631434));
#87750=CARTESIAN_POINT('Origin',(0.,0.,4.94191290631434));
#87751=CARTESIAN_POINT('Origin',(0.,0.,-8.86869034258935));
#87752=CARTESIAN_POINT('',(17.5762965073726,2.15247552586186E-15,-8.62202959520812));
#87753=CARTESIAN_POINT('',(-17.5762965073726,-2.15247552586187E-15,-8.6220295952081));
#87754=CARTESIAN_POINT('Origin',(0.,0.,-8.62202959520812));
#87755=CARTESIAN_POINT('Origin',(0.,0.,-8.62202959520812));
#87756=CARTESIAN_POINT('',(-16.6071946160828,-2.0337947729403E-15,-8.86869034258935));
#87757=CARTESIAN_POINT('',(-16.6071946160828,-2.0337947729403E-15,-8.86869034258935));
#87758=CARTESIAN_POINT('',(16.6071946160828,2.0337947729403E-15,-8.86869034258935));
#87759=CARTESIAN_POINT('Origin',(0.,0.,-8.86869034258935));
#87760=CARTESIAN_POINT('Origin',(0.,0.,-8.86869034258935));
#87761=CARTESIAN_POINT('Origin',(0.,0.,5.64211868066453));
#87762=CARTESIAN_POINT('',(-13.3064408708579,-1.62956902205396E-15,6.12666962630939));
#87763=CARTESIAN_POINT('Origin',(0.,0.,6.12666962630939));
#87764=CARTESIAN_POINT('',(-13.9143221901933,-1.70401301325252E-15,5.76544905435514));
#87765=CARTESIAN_POINT('Origin',(-13.4297712445485,-1.64467263679175E-15,
5.64211868066453));
#87766=CARTESIAN_POINT('',(13.9143221901933,1.92824426955719E-15,5.76544905435514));
#87767=CARTESIAN_POINT('Origin',(0.,0.,5.76544905435514));
#87768=CARTESIAN_POINT('Origin',(0.,0.,5.76544905435514));
#87769=CARTESIAN_POINT('Origin',(0.,0.,6.12666962630939));
#87770=CARTESIAN_POINT('',(12.4591576910941,1.54091037338483E-15,5.91101479760407));
#87771=CARTESIAN_POINT('',(-12.4591576910941,-1.52580675864705E-15,5.91101479760407));
#87772=CARTESIAN_POINT('Origin',(0.,0.,5.91101479760407));
#87773=CARTESIAN_POINT('Origin',(0.,0.,5.91101479760407));
#87774=CARTESIAN_POINT('',(-13.3064408708579,-1.62956902205396E-15,6.12666962630939));
#87775=CARTESIAN_POINT('Origin',(0.,0.,5.91101479760407));
#87776=CARTESIAN_POINT('',(12.4591576910941,-1.52580675864705E-15,5.91101479760407));
#87777=CARTESIAN_POINT('Origin',(0.,0.,5.03423736132904));
#87778=CARTESIAN_POINT('',(13.6758990082496,-1.71737624121704E-15,2.64803515038039));
#87779=CARTESIAN_POINT('',(13.0685506725942,-1.60043587506875E-15,5.03423736132904));
#87780=CARTESIAN_POINT('',(12.8785649144981,-4.62651215577902,2.6147440184906));
#87781=CARTESIAN_POINT('Origin',(-0.937114226824163,0.134736684811201,-1.03836599339337));
#87782=CARTESIAN_POINT('',(14.9513426147766,-4.92290433508688,-5.46532997546471));
#87783=CARTESIAN_POINT('Ctrl Pts',(12.8785649144981,-4.62651215577902,2.61474401849061));
#87784=CARTESIAN_POINT('Ctrl Pts',(13.278829444552,-4.68375292971506,1.05871968629378));
#87785=CARTESIAN_POINT('Ctrl Pts',(13.678412855787,-4.74088814688723,-0.497483831381018));
#87786=CARTESIAN_POINT('Ctrl Pts',(14.0774687012176,-4.79794842577841,-2.05382524940579));
#87787=CARTESIAN_POINT('Ctrl Pts',(14.3690279116768,-4.83963795382966,-3.19092342811977));
#87788=CARTESIAN_POINT('Ctrl Pts',(14.6603042032756,-4.8812871409245,-4.32809569652915));
#87789=CARTESIAN_POINT('Ctrl Pts',(14.9513426147766,-4.92290433508687,-5.46532997546471));
#87790=CARTESIAN_POINT('',(15.73602449803,-1.07552855510562E-15,-5.44596249471135));
#87791=CARTESIAN_POINT('Origin',(-1.07828029600555,0.155033301408076,-9.68767988915812));
#87792=CARTESIAN_POINT('',(13.0685506725942,-1.60043587506875E-15,5.03423736132904));
#87793=CARTESIAN_POINT('',(15.7326506103909,0.51121213621885,-5.46532997546471));
#87794=CARTESIAN_POINT('Origin',(-1.07828029600555,0.155033301408076,-9.68767988915812));
#87795=CARTESIAN_POINT('',(13.6603316446047,0.810794884002057,2.6147440184906));
#87796=CARTESIAN_POINT('Ctrl Pts',(15.7326506103909,0.511212136218851,-5.46532997546471));
#87797=CARTESIAN_POINT('Ctrl Pts',(15.3395296796034,0.568042178714901,-3.92886882847666));
#87798=CARTESIAN_POINT('Ctrl Pts',(14.9459770913082,0.624938443835918,-2.39252047018801));
#87799=CARTESIAN_POINT('Ctrl Pts',(14.5518755460098,0.681912741033039,-0.856315892565244));
#87800=CARTESIAN_POINT('Ctrl Pts',(14.2550284656633,0.724827197927523,0.30079158169481));
#87801=CARTESIAN_POINT('Ctrl Pts',(13.9578694621683,0.767785972485785,1.45781746616772));
#87802=CARTESIAN_POINT('Ctrl Pts',(13.6603316446047,0.810794884002048,2.61474401849061));
#87803=CARTESIAN_POINT('Origin',(-0.937114226824163,0.134736684811201,-1.03836599339337));
#87804=CARTESIAN_POINT('',(-12.8785649144981,-4.62651215577884,2.6147440184906));
#87805=CARTESIAN_POINT('',(-13.6603316446047,0.810794884002255,2.6147440184906));
#87806=CARTESIAN_POINT('Origin',(0.937114226824163,0.134736684811185,-1.03836599339337));
#87807=CARTESIAN_POINT('',(-15.7326506103909,0.511212136219076,-5.46532997546471));
#87808=CARTESIAN_POINT('Ctrl Pts',(-13.6603316446047,0.810794884002257,
2.61474401849061));
#87809=CARTESIAN_POINT('Ctrl Pts',(-14.0605092383751,0.752949454933123,
1.05871968629378));
#87810=CARTESIAN_POINT('Ctrl Pts',(-14.4600035646476,0.695194638237067,
-0.497483831381016));
#87811=CARTESIAN_POINT('Ctrl Pts',(-14.8589705815908,0.63751655140806,-2.05382524514076));
#87812=CARTESIAN_POINT('Ctrl Pts',(-15.1504648938438,0.595375638655163,
-3.19092342811977));
#87813=CARTESIAN_POINT('Ctrl Pts',(-15.4416763809839,0.553275726649975,
-4.32809569652915));
#87814=CARTESIAN_POINT('Ctrl Pts',(-15.7326506103909,0.51121213621909,-5.46532997546471));
#87815=CARTESIAN_POINT('',(-14.9513426147767,-4.92290433508666,-5.46532997546471));
#87816=CARTESIAN_POINT('Origin',(1.07828029600555,0.155033301408058,-9.68767988915812));
#87817=CARTESIAN_POINT('Ctrl Pts',(-14.9513426147767,-4.92290433508665,
-5.46532997546471));
#87818=CARTESIAN_POINT('Ctrl Pts',(-14.5221701265151,-4.86153458433446,
-3.78833599137146));
#87819=CARTESIAN_POINT('Ctrl Pts',(-14.0924827365919,-4.80009582568339,
-2.11147616269138));
#87820=CARTESIAN_POINT('Ctrl Pts',(-13.6621274936101,-4.73855928020904,
-0.434791406020226));
#87821=CARTESIAN_POINT('Ctrl Pts',(-13.4012014616513,-4.70124943702037,
0.58178898317796));
#87822=CARTESIAN_POINT('Ctrl Pts',(-13.1400290384343,-4.66390345000266,
1.59830486814573));
#87823=CARTESIAN_POINT('Ctrl Pts',(-12.8785649144981,-4.62651215577882,
2.6147440184906));
#87824=CARTESIAN_POINT('',(12.9587657595714,8.93577210236536,-5.46532997546471));
#87825=CARTESIAN_POINT('',(15.2393928192273,3.94189542962978,-5.46532997546471));
#87826=CARTESIAN_POINT('Origin',(-0.990924439240726,-0.452540028181473,
-9.68767988916879));
#87827=CARTESIAN_POINT('',(11.0534534467936,8.06741692762184,2.6147440184906));
#87828=CARTESIAN_POINT('Ctrl Pts',(12.9587657595714,8.93577210236537,-5.46532997546471));
#87829=CARTESIAN_POINT('Ctrl Pts',(12.5973267470854,8.77104335500624,-3.92886882847666));
#87830=CARTESIAN_POINT('Ctrl Pts',(12.235488798542,8.60613694599651,-2.39252047018801));
#87831=CARTESIAN_POINT('Ctrl Pts',(11.8731468506549,8.44099939318352,-0.856315892565245));
#87832=CARTESIAN_POINT('Ctrl Pts',(11.6002218885467,8.3166136834777,0.300791581694808));
#87833=CARTESIAN_POINT('Ctrl Pts',(11.3270105600498,8.19209661777709,1.45781746616771));
#87834=CARTESIAN_POINT('Ctrl Pts',(11.0534534467936,8.06741692762186,2.6147440184906));
#87835=CARTESIAN_POINT('',(13.3354195459858,3.07060816729373,2.6147440184906));
#87836=CARTESIAN_POINT('Origin',(-0.861194805452217,-0.393294489564575,
-1.03836599340818));
#87837=CARTESIAN_POINT('Ctrl Pts',(13.3354195459858,3.07060816729374,2.61474401849061));
#87838=CARTESIAN_POINT('Ctrl Pts',(13.7030901947733,3.23885350672491,1.05871968629378));
#87839=CARTESIAN_POINT('Ctrl Pts',(14.0701307816529,3.40681940552155,-0.49748383138102));
#87840=CARTESIAN_POINT('Ctrl Pts',(14.4366870362378,3.57456312234433,-2.05382524514076));
#87841=CARTESIAN_POINT('Ctrl Pts',(14.7045013135956,3.6971204699282,-3.19092342811977));
#87842=CARTESIAN_POINT('Ctrl Pts',(14.9720557734904,3.81955879654057,-4.32809569652915));
#87843=CARTESIAN_POINT('Ctrl Pts',(15.2393928192273,3.94189542962981,-5.46532997546471));
#87844=CARTESIAN_POINT('',(-15.2393928192272,3.94189542963,-5.46532997546471));
#87845=CARTESIAN_POINT('',(-12.9587657595713,8.93577210236555,-5.46532997546471));
#87846=CARTESIAN_POINT('Origin',(0.990924439244865,-0.452540028182586,-9.68767988916981));
#87847=CARTESIAN_POINT('',(-13.3354195459858,3.07060816729392,2.6147440184906));
#87848=CARTESIAN_POINT('Ctrl Pts',(-15.2393928192272,3.94189542963002,-5.46532997546471));
#87849=CARTESIAN_POINT('Ctrl Pts',(-14.8782069215336,3.77661243818618,-3.92886882847666));
#87850=CARTESIAN_POINT('Ctrl Pts',(-14.5166255085638,3.61114429462567,-2.39252047018801));
#87851=CARTESIAN_POINT('Ctrl Pts',(-14.154539359383,3.44544662077634,-0.856315892565249));
#87852=CARTESIAN_POINT('Ctrl Pts',(-13.8818070712189,3.32063901398268,0.300791581694806));
#87853=CARTESIAN_POINT('Ctrl Pts',(-13.6087879807142,3.19570100579582,1.45781746616771));
#87854=CARTESIAN_POINT('Ctrl Pts',(-13.3354195459858,3.07060816729395,2.6147440184906));
#87855=CARTESIAN_POINT('',(-11.0534534467934,8.06741692762199,2.6147440184906));
#87856=CARTESIAN_POINT('Origin',(0.861194805416237,-0.393294489547195,-1.03836599339796));
#87857=CARTESIAN_POINT('Ctrl Pts',(-11.0534534467934,8.06741692762199,2.6147440184906));
#87858=CARTESIAN_POINT('Ctrl Pts',(-11.4213778613707,8.23510659748291,1.05871968629378));
#87859=CARTESIAN_POINT('Ctrl Pts',(-11.788678486004,8.40250309302417,-0.497483831381018));
#87860=CARTESIAN_POINT('Ctrl Pts',(-12.1554940265031,8.56967905289034,-2.05382524514076));
#87861=CARTESIAN_POINT('Ctrl Pts',(-12.4234977440052,8.69182158442034,-3.19092342811977));
#87862=CARTESIAN_POINT('Ctrl Pts',(-12.6912413672041,8.81384570117397,-4.32809569652915));
#87863=CARTESIAN_POINT('Ctrl Pts',(-12.9587657595713,8.93577210236556,-5.46532997546471));
#87864=CARTESIAN_POINT('',(-2.74499836100712,15.4997618392967,-5.46532997546471));
#87865=CARTESIAN_POINT('',(2.74499836100712,15.4997618392967,-5.46532997546471));
#87866=CARTESIAN_POINT('Origin',(-9.82547376793264E-14,-1.08936849638624,
-9.68767988911357));
#87867=CARTESIAN_POINT('',(-2.74661004991401,13.4059010222448,2.6147440184906));
#87868=CARTESIAN_POINT('Ctrl Pts',(-2.74499836100712,15.4997618392967,-5.46532997546471));
#87869=CARTESIAN_POINT('Ctrl Pts',(-2.74530301392585,15.1025545544441,-3.92886882847666));
#87870=CARTESIAN_POINT('Ctrl Pts',(-2.7456117841503,14.7049105812728,-2.39252047018801));
#87871=CARTESIAN_POINT('Ctrl Pts',(-2.74591966746971,14.3067121335667,-0.856315892565247));
#87872=CARTESIAN_POINT('Ctrl Pts',(-2.74615157283914,14.0067791644875,0.300791581694806));
#87873=CARTESIAN_POINT('Ctrl Pts',(-2.74638295349,13.7065311401264,1.45781746616772));
#87874=CARTESIAN_POINT('Ctrl Pts',(-2.746610049914,13.4059010222448,2.61474401849061));
#87875=CARTESIAN_POINT('',(2.74661004991401,13.4059010222448,2.6147440184906));
#87876=CARTESIAN_POINT('Origin',(-3.71924713249427E-14,-0.94675078472652,
-1.03836599339739));
#87877=CARTESIAN_POINT('Ctrl Pts',(2.746610049914,13.4059010222448,2.61474401849061));
#87878=CARTESIAN_POINT('Ctrl Pts',(2.74630461344459,13.8102376480019,1.05871968629378));
#87879=CARTESIAN_POINT('Ctrl Pts',(2.7459916279415,14.2138850654537,-0.497483831381017));
#87880=CARTESIAN_POINT('Ctrl Pts',(2.74567954736412,14.6169996210264,-2.05382524514076));
#87881=CARTESIAN_POINT('Ctrl Pts',(2.74545153424673,14.9115242186639,-3.19092342811977));
#87882=CARTESIAN_POINT('Ctrl Pts',(2.74522385433836,15.2057630349255,-4.32809569652915));
#87883=CARTESIAN_POINT('Ctrl Pts',(2.74499836100712,15.4997618392967,-5.46532997546471));
#87884=CARTESIAN_POINT('',(6.07056434235145,14.5232875631595,-5.46532997546471));
#87885=CARTESIAN_POINT('',(10.6890434799775,11.5551712475411,-5.46532997546471));
#87886=CARTESIAN_POINT('Origin',(-0.588957074466897,-0.916435096252204,
-9.68767988914712));
#87887=CARTESIAN_POINT('',(4.93718187959547,12.7626910983658,2.6147440184906));
#87888=CARTESIAN_POINT('Ctrl Pts',(6.07056434235145,14.5232875631595,-5.46532997546471));
#87889=CARTESIAN_POINT('Ctrl Pts',(5.85556158082525,14.189300239314,-3.92886882847666));
#87890=CARTESIAN_POINT('Ctrl Pts',(5.64031926407142,13.8549477758611,-2.39252047018801));
#87891=CARTESIAN_POINT('Ctrl Pts',(5.4247779218639,13.5201283792499,-0.856315892565248));
#87892=CARTESIAN_POINT('Ctrl Pts',(5.26242682506772,13.267934086908,0.300791581694809));
#87893=CARTESIAN_POINT('Ctrl Pts',(5.09990583794776,13.0154744695129,1.45781746616771));
#87894=CARTESIAN_POINT('Ctrl Pts',(4.93718187959545,12.7626910983658,2.6147440184906));
#87895=CARTESIAN_POINT('',(9.55837269519504,9.79283209313127,2.6147440184906));
#87896=CARTESIAN_POINT('Origin',(-0.511852118179011,-0.796457442358354,
-1.03836599339643));
#87897=CARTESIAN_POINT('Ctrl Pts',(9.55837269519502,9.79283209313128,2.6147440184906));
#87898=CARTESIAN_POINT('Ctrl Pts',(9.77671662956264,10.133146839425,1.05871968629378));
#87899=CARTESIAN_POINT('Ctrl Pts',(9.99468159913746,10.4728858681128,-0.497483831381017));
#87900=CARTESIAN_POINT('Ctrl Pts',(10.2123592431023,10.8121761356224,-2.05382524514076));
#87901=CARTESIAN_POINT('Ctrl Pts',(10.3713994454892,11.0600692670888,-3.19092342811977));
#87902=CARTESIAN_POINT('Ctrl Pts',(10.5302854231128,11.3077218038168,-4.32809569652915));
#87903=CARTESIAN_POINT('Ctrl Pts',(10.6890434799775,11.5551712475411,-5.46532997546471));
#87904=CARTESIAN_POINT('',(-10.6890434799774,11.5551712475413,-5.46532997546471));
#87905=CARTESIAN_POINT('',(-6.07056434235124,14.5232875631596,-5.46532997546471));
#87906=CARTESIAN_POINT('Origin',(0.588957074505134,-0.916435096306598,-9.6876798891643));
#87907=CARTESIAN_POINT('',(-9.55837269519489,9.79283209313141,2.6147440184906));
#87908=CARTESIAN_POINT('Ctrl Pts',(-10.6890434799774,11.5551712475413,-5.46532997546471));
#87909=CARTESIAN_POINT('Ctrl Pts',(-10.4745532991395,11.2208545080897,-3.92886882847666));
#87910=CARTESIAN_POINT('Ctrl Pts',(-10.25983049047,10.8861681770637,-2.39252047018801));
#87911=CARTESIAN_POINT('Ctrl Pts',(-10.0448071641228,10.5510158718736,-0.856315892565248));
#87912=CARTESIAN_POINT('Ctrl Pts',(-9.88284624974924,10.2985708245147,0.300791581694807));
#87913=CARTESIAN_POINT('Ctrl Pts',(-9.72071456220919,10.0458610194711,1.45781746616771));
#87914=CARTESIAN_POINT('Ctrl Pts',(-9.55837269519489,9.79283209313141,2.6147440184906));
#87915=CARTESIAN_POINT('',(-4.93718187959529,12.7626910983659,2.6147440184906));
#87916=CARTESIAN_POINT('Origin',(0.511852118212275,-0.796457442409964,-1.03836599341197));
#87917=CARTESIAN_POINT('Ctrl Pts',(-4.93718187959529,12.7626910983659,2.61474401849061));
#87918=CARTESIAN_POINT('Ctrl Pts',(-5.15603971298079,13.1026755818146,1.05871968629378));
#87919=CARTESIAN_POINT('Ctrl Pts',(-5.374531282876,13.4420761850259,-0.497483831381019));
#87920=CARTESIAN_POINT('Ctrl Pts',(-5.59273400461729,13.7810290055386,-2.05382524514076));
#87921=CARTESIAN_POINT('Ctrl Pts',(-5.75215784068531,14.0286755906086,-3.19092342811977));
#87922=CARTESIAN_POINT('Ctrl Pts',(-5.91142689136349,14.2760819412331,-4.32809569652915));
#87923=CARTESIAN_POINT('Ctrl Pts',(-6.07056434235125,14.5232875631596,-5.46532997546471));
#87924=CARTESIAN_POINT('',(13.5115300540086,-8.07565407112479,-5.46532997546471));
#87925=CARTESIAN_POINT('',(9.9163467712731,-12.2247167569933,-5.46532997546471));
#87926=CARTESIAN_POINT('Origin',(-0.823289777622591,0.713384653218671,-9.68767988916813));
#87927=CARTESIAN_POINT('',(11.9301510645449,-6.70324880648548,2.6147440184906));
#87928=CARTESIAN_POINT('Ctrl Pts',(13.5115300540086,-8.07565407112482,-5.46532997546471));
#87929=CARTESIAN_POINT('Ctrl Pts',(13.2115403227848,-7.81530837572417,-3.92886882847666));
#87930=CARTESIAN_POINT('Ctrl Pts',(12.9112232608118,-7.55467359863853,-2.39252047018801));
#87931=CARTESIAN_POINT('Ctrl Pts',(12.6104865741459,-7.29367638823024,-0.856315892565246));
#87932=CARTESIAN_POINT('Ctrl Pts',(12.3839642261499,-7.09708680158041,0.300791581694807));
#87933=CARTESIAN_POINT('Ctrl Pts',(12.1572034316412,-6.90029129415331,1.45781746616771));
#87934=CARTESIAN_POINT('Ctrl Pts',(11.9301510645449,-6.70324880648547,2.6147440184906));
#87935=CARTESIAN_POINT('',(8.33285691824855,-10.8547475587647,2.6147440184906));
#87936=CARTESIAN_POINT('Origin',(-0.715506502546432,0.619989913722224,-1.0383659933872));
#87937=CARTESIAN_POINT('Ctrl Pts',(8.33285691824854,-10.8547475587647,2.6147440184906));
#87938=CARTESIAN_POINT('Ctrl Pts',(8.63863416941083,-11.1193009047872,1.05871968629378));
#87939=CARTESIAN_POINT('Ctrl Pts',(8.94389549525559,-11.3833972101742,-0.497483831381018));
#87940=CARTESIAN_POINT('Ctrl Pts',(9.24875351836159,-11.647145249137,-2.05382524514076));
#87941=CARTESIAN_POINT('Ctrl Pts',(9.47148967450035,-11.8398455224944,-3.19092342811977));
#87942=CARTESIAN_POINT('Ctrl Pts',(9.69400963328047,-12.0323589006728,-4.32809569652915));
#87943=CARTESIAN_POINT('Ctrl Pts',(9.91634677127309,-12.2247167569933,-5.46532997546471));
#87944=CARTESIAN_POINT('',(-1.73298089344877,-15.6452679842754,-5.46532997546471));
#87945=CARTESIAN_POINT('',(-7.00059417338805,-14.0985571707312,-5.46532997546471));
#87946=CARTESIAN_POINT('Origin',(0.306910571885848,1.04524141815081,-9.68767988916436));
#87947=CARTESIAN_POINT('',(-1.14152572760881,-13.6366773078239,2.6147440184906));
#87948=CARTESIAN_POINT('Ctrl Pts',(-1.73298089344877,-15.6452679842754,
-5.46532997546471));
#87949=CARTESIAN_POINT('Ctrl Pts',(-1.62078235715629,-15.2642362160366,
-3.92886882847666));
#87950=CARTESIAN_POINT('Ctrl Pts',(-1.5084568410213,-14.8827866084033,-2.39252047018801));
#87951=CARTESIAN_POINT('Ctrl Pts',(-1.3959759623371,-14.5008047364799,-0.856315892565247));
#87952=CARTESIAN_POINT('Ctrl Pts',(-1.31125256850485,-14.2130864953857,
0.300791581694806));
#87953=CARTESIAN_POINT('Ctrl Pts',(-1.2264409168063,-13.925065813132,1.45781746616772));
#87954=CARTESIAN_POINT('Ctrl Pts',(-1.14152572760881,-13.6366773078239,
2.61474401849061));
#87955=CARTESIAN_POINT('',(-6.4122318159117,-12.0890583638066,2.6147440184906));
#87956=CARTESIAN_POINT('Origin',(0.266730519261321,0.908400725671796,-1.03836599338752));
#87957=CARTESIAN_POINT('Ctrl Pts',(-6.4122318159117,-12.0890583638066,2.61474401849061));
#87958=CARTESIAN_POINT('Ctrl Pts',(-6.5258535431646,-12.477102566593,1.05871968629378));
#87959=CARTESIAN_POINT('Ctrl Pts',(-6.63927385475469,-12.8644876056617,
-0.497483831381018));
#87960=CARTESIAN_POINT('Ctrl Pts',(-6.75254491007499,-13.2513611125545,
-2.05382524514076));
#87961=CARTESIAN_POINT('Ctrl Pts',(-6.83530330103606,-13.5340196332628,
-3.19092342811977));
#87962=CARTESIAN_POINT('Ctrl Pts',(-6.91798149779113,-13.8164038548732,
-4.32809569652915));
#87963=CARTESIAN_POINT('Ctrl Pts',(-7.00059417338803,-14.0985571707312,
-5.46532997546471));
#87964=CARTESIAN_POINT('',(-9.91634677127328,-12.2247167569932,-5.46532997546471));
#87965=CARTESIAN_POINT('',(-13.5115300540087,-8.07565407112461,-5.46532997546471));
#87966=CARTESIAN_POINT('Origin',(0.823289777498141,0.713384653116,-9.68767988912725));
#87967=CARTESIAN_POINT('',(-8.33285691824872,-10.8547475587646,2.61474401849061));
#87968=CARTESIAN_POINT('Ctrl Pts',(-9.91634677127329,-12.2247167569932,
-5.46532997546471));
#87969=CARTESIAN_POINT('Ctrl Pts',(-9.61595802958152,-11.9648315442198,
-3.92886882847666));
#87970=CARTESIAN_POINT('Ctrl Pts',(-9.31523656461692,-11.7046634730656,
-2.39252047018801));
#87971=CARTESIAN_POINT('Ctrl Pts',(-9.01409663655801,-11.4441316280326,
-0.856315892565249));
#87972=CARTESIAN_POINT('Ctrl Pts',(-8.78727055712117,-11.2478925661512,
0.300791581694807));
#87973=CARTESIAN_POINT('Ctrl Pts',(-8.56020671840674,-11.0514467903809,
1.45781746616772));
#87974=CARTESIAN_POINT('Ctrl Pts',(-8.3328569182487,-10.8547475587646,2.61474401849061));
#87975=CARTESIAN_POINT('',(-11.930151064545,-6.70324880648531,2.61474401849061));
#87976=CARTESIAN_POINT('Origin',(0.715506502489277,0.619989913672336,-1.03836599336785));
#87977=CARTESIAN_POINT('Ctrl Pts',(-11.930151064545,-6.70324880648531,2.61474401849061));
#87978=CARTESIAN_POINT('Ctrl Pts',(-12.2355282790063,-6.96826381947133,
1.05871968629378));
#87979=CARTESIAN_POINT('Ctrl Pts',(-12.5403796810185,-7.23283320217974,
-0.49748383138102));
#87980=CARTESIAN_POINT('Ctrl Pts',(-12.8448289654926,-7.49705295066959,
-2.05382524514076));
#87981=CARTESIAN_POINT('Ctrl Pts',(-13.0672664879565,-7.69009786565978,
-3.19092342811977));
#87982=CARTESIAN_POINT('Ctrl Pts',(-13.2894882494729,-7.88295538182595,
-4.32809569652915));
#87983=CARTESIAN_POINT('Ctrl Pts',(-13.5115300540087,-8.07565407112462,
-5.46532997546471));
#87984=CARTESIAN_POINT('',(7.00059417338784,-14.0985571707313,-5.46532997546471));
#87985=CARTESIAN_POINT('',(1.73298089344855,-15.6452679842754,-5.46532997546471));
#87986=CARTESIAN_POINT('Origin',(-0.306910571834217,1.04524141797904,-9.68767988911857));
#87987=CARTESIAN_POINT('',(6.41223181591152,-12.0890583638067,2.6147440184906));
#87988=CARTESIAN_POINT('Ctrl Pts',(7.00059417338784,-14.0985571707313,-5.46532997546471));
#87989=CARTESIAN_POINT('Ctrl Pts',(6.88898026176519,-13.717353741201,-3.92886882847666));
#87990=CARTESIAN_POINT('Ctrl Pts',(6.77724727135186,-13.3357301523181,-2.39252047018801));
#87991=CARTESIAN_POINT('Ctrl Pts',(6.665357216431,-12.9535747988851,-0.856315892565249));
#87992=CARTESIAN_POINT('Ctrl Pts',(6.58107884574378,-12.6657258872056,0.300791581694807));
#87993=CARTESIAN_POINT('Ctrl Pts',(6.4967112102627,-12.3775748300272,1.45781746616771));
#87994=CARTESIAN_POINT('Ctrl Pts',(6.41223181591153,-12.0890583638067,2.6147440184906));
#87995=CARTESIAN_POINT('',(1.14152572760861,-13.6366773078239,2.6147440184906));
#87996=CARTESIAN_POINT('Origin',(-0.266730519284407,0.908400725745018,-1.03836599340707));
#87997=CARTESIAN_POINT('Ctrl Pts',(1.14152572760862,-13.6366773078239,2.6147440184906));
#87998=CARTESIAN_POINT('Ctrl Pts',(1.2557335831541,-14.0245494078154,1.05871968629378));
#87999=CARTESIAN_POINT('Ctrl Pts',(1.36975450952629,-14.411758090472,-0.497483831381019));
#88000=CARTESIAN_POINT('Ctrl Pts',(1.48362444308898,-14.7984557508468,-2.05382524514076));
#88001=CARTESIAN_POINT('Ctrl Pts',(1.56682038801811,-15.080985794118,-3.19092342811977));
#88002=CARTESIAN_POINT('Ctrl Pts',(1.6499354993178,-15.3632417260429,-4.32809569652915));
#88003=CARTESIAN_POINT('Ctrl Pts',(1.73298089344855,-15.6452679842754,-5.46532997546471));
#88004=CARTESIAN_POINT('Origin',(0.,0.,-8.62202959520812));
#88005=CARTESIAN_POINT('',(16.7057269056484,-5.55111512312578E-16,-5.20166110736635));
#88006=CARTESIAN_POINT('',(17.5762965073726,-2.15247552586187E-15,-8.62202959520812));
#88007=CARTESIAN_POINT('',(16.0018747190063,-4.80108026882922,-5.20507760384135));
#88008=CARTESIAN_POINT('Origin',(-1.14472725656124,0.164586932037927,-9.70476622209448));
#88009=CARTESIAN_POINT('',(13.9356166188379,-4.51728618677704,2.87709523867187));
#88010=CARTESIAN_POINT('Ctrl Pts',(16.0018747190063,-4.80108026882921,-5.20507760384135));
#88011=CARTESIAN_POINT('Ctrl Pts',(15.6318627383349,-4.74997519723103,-3.75496347264913));
#88012=CARTESIAN_POINT('Ctrl Pts',(15.2615370048954,-4.69896135726135,-2.30492612391988));
#88013=CARTESIAN_POINT('Ctrl Pts',(14.8908189592186,-4.64805794703302,-0.854985236809349));
#88014=CARTESIAN_POINT('Ctrl Pts',(14.5727290602808,-4.60438092401258,0.389118080051586));
#88015=CARTESIAN_POINT('Ctrl Pts',(14.2543502786107,-4.56078522296996,1.63315045290804));
#88016=CARTESIAN_POINT('Ctrl Pts',(13.9356166188379,-4.51728618677703,2.87709523867187));
#88017=CARTESIAN_POINT('',(14.6456014158681,-9.0205620750794E-16,2.89233653772541));
#88018=CARTESIAN_POINT('Origin',(-1.00356118737986,0.144290315441051,-1.05545232632974));
#88019=CARTESIAN_POINT('',(17.5762965073726,-2.15247552586187E-15,-8.62202959520812));
#88020=CARTESIAN_POINT('',(14.6437928161456,0.408187454831152,2.87709523867187));
#88021=CARTESIAN_POINT('Origin',(-1.00356118737986,0.144290315441051,-1.05545232632974));
#88022=CARTESIAN_POINT('',(16.7063069772842,0.0983537048588373,-5.20507760384135));
#88023=CARTESIAN_POINT('Ctrl Pts',(14.6437928161456,0.408187454831128,2.87709523867187));
#88024=CARTESIAN_POINT('Ctrl Pts',(15.0641690510667,0.344669830214016,1.23307977231272));
#88025=CARTESIAN_POINT('Ctrl Pts',(15.4839997756004,0.281487984625945,-0.411088229465956));
#88026=CARTESIAN_POINT('Ctrl Pts',(15.9034155138528,0.218567936571954,-2.05537199759547));
#88027=CARTESIAN_POINT('Ctrl Pts',(16.1712077467516,0.178394193372236,-3.1052286949651));
#88028=CARTESIAN_POINT('Ctrl Pts',(16.4388297533631,0.138327718067133,-4.15513295741812));
#88029=CARTESIAN_POINT('Ctrl Pts',(16.7063069772842,0.0983537048588252,
-5.20507760384135));
#88030=CARTESIAN_POINT('Origin',(-1.14472725656124,0.164586932037927,-9.70476622209448));
#88031=CARTESIAN_POINT('',(-14.6437928161456,0.408187454831364,2.87709523867187));
#88032=CARTESIAN_POINT('',(-13.935616618838,-4.51728618677683,2.87709523867187));
#88033=CARTESIAN_POINT('Origin',(1.00356118737986,0.144290315441036,-1.05545232632974));
#88034=CARTESIAN_POINT('',(-16.0018747190064,-4.80108026882899,-5.20507760384135));
#88035=CARTESIAN_POINT('Ctrl Pts',(-13.935616618838,-4.51728618677684,2.87709523867187));
#88036=CARTESIAN_POINT('Ctrl Pts',(-14.3568596453072,-4.57477514375573,
1.23307977231272));
#88037=CARTESIAN_POINT('Ctrl Pts',(-14.7774846585082,-4.63243259031745,
-0.411088229465949));
#88038=CARTESIAN_POINT('Ctrl Pts',(-15.1976377383996,-4.69022431462755,
-2.05537199759547));
#88039=CARTESIAN_POINT('Ctrl Pts',(-15.4659007556441,-4.72712368078047,
-3.1052286949651));
#88040=CARTESIAN_POINT('Ctrl Pts',(-15.7339702211038,-4.76407801143741,
-4.15513295741812));
#88041=CARTESIAN_POINT('Ctrl Pts',(-16.0018747190064,-4.80108026882899,
-5.20507760384135));
#88042=CARTESIAN_POINT('',(-16.7063069772842,0.0983537048590811,-5.20507760384135));
#88043=CARTESIAN_POINT('Origin',(1.14472725656124,0.164586932037911,-9.70476622209449));
#88044=CARTESIAN_POINT('Ctrl Pts',(-16.7063069772842,0.0983537048590963,
-5.20507760384135));
#88045=CARTESIAN_POINT('Ctrl Pts',(-16.3368851191879,0.153563169121086,
-3.75496347264913));
#88046=CARTESIAN_POINT('Ctrl Pts',(-15.9671879204351,0.208948563859175,
-2.30492612391988));
#88047=CARTESIAN_POINT('Ctrl Pts',(-15.5971454125005,0.264550442287883,
-0.854985236809342));
#88048=CARTESIAN_POINT('Ctrl Pts',(-15.2796351501211,0.312258926124563,
0.389118080051595));
#88049=CARTESIAN_POINT('Ctrl Pts',(-14.9618706178388,0.360126825498279,
1.63315045290804));
#88050=CARTESIAN_POINT('Ctrl Pts',(-14.6437928161456,0.40818745483137,2.87709523867187));
#88051=CARTESIAN_POINT('',(10.8659736780762,-12.6901923664643,-5.20507760384135));
#88052=CARTESIAN_POINT('',(14.1074137925972,-8.94937105918356,-5.20507760384135));
#88053=CARTESIAN_POINT('Origin',(-0.874023435400204,0.757345617923459,-9.70476622215003));
#88054=CARTESIAN_POINT('',(9.28115741607829,-11.334346123992,2.87709523867187));
#88055=CARTESIAN_POINT('Ctrl Pts',(10.8659736780762,-12.6901923664643,-5.20507760384135));
#88056=CARTESIAN_POINT('Ctrl Pts',(10.5513660696195,-12.4206261621453,-3.59666600951091));
#88057=CARTESIAN_POINT('Ctrl Pts',(10.2363736133453,-12.1509459082059,-1.9883487212344));
#88058=CARTESIAN_POINT('Ctrl Pts',(9.92089023043911,-11.8811150096239,-0.380153053637523));
#88059=CARTESIAN_POINT('Ctrl Pts',(9.70788468030107,-11.6989327391434,0.705655649662519));
#88060=CARTESIAN_POINT('Ctrl Pts',(9.49465478510907,-11.5166815848276,1.79140883582473));
#88061=CARTESIAN_POINT('Ctrl Pts',(9.28115741607828,-11.334346123992,2.87709523867188));
#88062=CARTESIAN_POINT('',(12.5398252398854,-7.5736429803373,2.87709523867187));
#88063=CARTESIAN_POINT('Origin',(-0.766240160099769,0.663950878237602,-1.05545232629423));
#88064=CARTESIAN_POINT('Ctrl Pts',(12.5398252398854,-7.57364298033732,2.87709523867187));
#88065=CARTESIAN_POINT('Ctrl Pts',(12.8591280121352,-7.85434995773017,1.23307977231272));
#88066=CARTESIAN_POINT('Ctrl Pts',(13.1781534076931,-8.13447953464675,-0.411088229465952));
#88067=CARTESIAN_POINT('Ctrl Pts',(13.4969712330088,-8.41416451494068,-2.05537199759547));
#88068=CARTESIAN_POINT('Ctrl Pts',(13.7005328296359,-8.59274023003717,-3.10522869496511));
#88069=CARTESIAN_POINT('Ctrl Pts',(13.9040092161996,-8.77113367435921,-4.15513295741812));
#88070=CARTESIAN_POINT('Ctrl Pts',(14.1074137925972,-8.94937105918357,-5.20507760384135));
#88071=CARTESIAN_POINT('',(-7.02951640698345,-15.1557337451693,-5.20507760384135));
#88072=CARTESIAN_POINT('',(-2.28020276965841,-16.5502580523615,-5.20507760384135));
#88073=CARTESIAN_POINT('Origin',(0.325823348666811,1.10965242068313,-9.70476622200136));
#88074=CARTESIAN_POINT('',(-6.45455175213294,-13.1508952820527,2.87709523867187));
#88075=CARTESIAN_POINT('Ctrl Pts',(-7.02951640698346,-15.1557337451693,
-5.20507760384135));
#88076=CARTESIAN_POINT('Ctrl Pts',(-6.91686081367391,-14.7640340059215,
-3.62275895686273));
#88077=CARTESIAN_POINT('Ctrl Pts',(-6.80425954802681,-14.3719495108703,
-2.04053160694041));
#88078=CARTESIAN_POINT('Ctrl Pts',(-6.69172285615924,-13.9793742084975,
-0.458421487187023));
#88079=CARTESIAN_POINT('Ctrl Pts',(-6.61263250329852,-13.7034738006056,
0.653479400952417));
#88080=CARTESIAN_POINT('Ctrl Pts',(-6.53357407923927,-13.4273304491785,
1.76532233007841));
#88081=CARTESIAN_POINT('Ctrl Pts',(-6.45455175213295,-13.1508952820527,
2.87709523867187));
#88082=CARTESIAN_POINT('',(-1.67999631123863,-14.5528312515023,2.87709523867187));
#88083=CARTESIAN_POINT('Origin',(0.285643296086849,0.972811728362482,-1.05545232626613));
#88084=CARTESIAN_POINT('Ctrl Pts',(-1.6799963112386,-14.5528312515023,2.87709523867187));
#88085=CARTESIAN_POINT('Ctrl Pts',(-1.8026931939087,-14.9598891620095,1.23307977231273));
#88086=CARTESIAN_POINT('Ctrl Pts',(-1.92498008107355,-15.3664549009767,
-0.41108822946595));
#88087=CARTESIAN_POINT('Ctrl Pts',(-2.04694877672028,-15.7726471352984,
-2.05537199759547));
#88088=CARTESIAN_POINT('Ctrl Pts',(-2.12482441745583,-16.0319963096245,
-3.1052286949651));
#88089=CARTESIAN_POINT('Ctrl Pts',(-2.20256965640269,-16.2911922561345,
-4.15513295741812));
#88090=CARTESIAN_POINT('Ctrl Pts',(-2.28020276965841,-16.5502580523615,
-5.20507760384135));
#88091=CARTESIAN_POINT('',(-14.1074137925973,-8.94937105918337,-5.20507760384135));
#88092=CARTESIAN_POINT('',(-10.8659736780764,-12.6901923664641,-5.20507760384135));
#88093=CARTESIAN_POINT('Origin',(0.874023435123159,0.757345617689386,-9.70476622205794));
#88094=CARTESIAN_POINT('',(-12.5398252398855,-7.57364298033712,2.87709523867187));
#88095=CARTESIAN_POINT('Ctrl Pts',(-14.1074137925973,-8.94937105918338,
-5.20507760384135));
#88096=CARTESIAN_POINT('Ctrl Pts',(-13.8264848392586,-8.70320136698007,
-3.75496347264913));
#88097=CARTESIAN_POINT('Ctrl Pts',(-13.5454193698163,-8.4567348122447,-2.30492612391989));
#88098=CARTESIAN_POINT('Ctrl Pts',(-13.2641804477244,-8.20989945160143,
-0.854985236809355));
#88099=CARTESIAN_POINT('Ctrl Pts',(-13.0228669714886,-7.99810551322451,
0.389118080051585));
#88100=CARTESIAN_POINT('Ctrl Pts',(-12.781425776345,-7.7860399972756,1.63315045290803));
#88101=CARTESIAN_POINT('Ctrl Pts',(-12.5398252398854,-7.57364298033715,
2.87709523867186));
#88102=CARTESIAN_POINT('',(-9.28115741607846,-11.3343461239919,2.87709523867187));
#88103=CARTESIAN_POINT('Origin',(0.766240160049487,0.66395087819444,-1.05545232627727));
#88104=CARTESIAN_POINT('Ctrl Pts',(-9.28115741607846,-11.3343461239919,
2.87709523867187));
#88105=CARTESIAN_POINT('Ctrl Pts',(-9.60444872358046,-11.610450086327,1.23307977231272));
#88106=CARTESIAN_POINT('Ctrl Pts',(-9.92712903289141,-11.8863616679203,
-0.411088229465947));
#88107=CARTESIAN_POINT('Ctrl Pts',(-10.2493397311838,-12.1621310652273,
-2.05537200053958));
#88108=CARTESIAN_POINT('Ctrl Pts',(-10.4550676381112,-12.3382067238051,
-3.1052286949651));
#88109=CARTESIAN_POINT('Ctrl Pts',(-10.6606030034384,-12.5142239799647,
-4.15513295741812));
#88110=CARTESIAN_POINT('Ctrl Pts',(-10.8659736780764,-12.6901923664641,
-5.20507760384135));
#88111=CARTESIAN_POINT('',(2.28020276965817,-16.5502580523615,-5.20507760384135));
#88112=CARTESIAN_POINT('',(7.02951640698323,-15.1557337451694,-5.20507760384135));
#88113=CARTESIAN_POINT('Origin',(-0.325823348773507,1.10965242105334,-9.70476622209937));
#88114=CARTESIAN_POINT('',(1.67999631123842,-14.5528312515024,2.87709523867187));
#88115=CARTESIAN_POINT('Ctrl Pts',(2.28020276965818,-16.5502580523615,-5.20507760384135));
#88116=CARTESIAN_POINT('Ctrl Pts',(2.17298104614731,-16.1924535020959,-3.75496347264914));
#88117=CARTESIAN_POINT('Ctrl Pts',(2.06554599781792,-15.8344014512619,-2.30492612391988));
#88118=CARTESIAN_POINT('Ctrl Pts',(1.95784752666939,-15.4760384148371,-0.854985236809349));
#88119=CARTESIAN_POINT('Ctrl Pts',(1.86543822476761,-15.1685495742783,0.389118080051586));
#88120=CARTESIAN_POINT('Ctrl Pts',(1.77283494356892,-14.8608317391138,1.63315045290804));
#88121=CARTESIAN_POINT('Ctrl Pts',(1.67999631123846,-14.5528312515024,2.87709523867186));
#88122=CARTESIAN_POINT('',(6.45455175213275,-13.1508952820528,2.87709523867187));
#88123=CARTESIAN_POINT('Origin',(-0.285643296179897,0.972811728678056,-1.05545232634991));
#88124=CARTESIAN_POINT('Ctrl Pts',(6.45455175213274,-13.1508952820528,2.87709523867187));
#88125=CARTESIAN_POINT('Ctrl Pts',(6.57140468760753,-13.5596691302799,1.23307977231272));
#88126=CARTESIAN_POINT('Ctrl Pts',(6.68833644522585,-13.967807277155,-0.41108822946595));
#88127=CARTESIAN_POINT('Ctrl Pts',(6.80533395090074,-14.375459185214,-2.05537200005118));
#88128=CARTESIAN_POINT('Ctrl Pts',(6.88003554244981,-14.635740343811,-3.1052286949651));
#88129=CARTESIAN_POINT('Ctrl Pts',(6.95476399392733,-14.8958220990456,-4.15513295741812));
#88130=CARTESIAN_POINT('Ctrl Pts',(7.02951640698322,-15.1557337451694,-5.20507760384135));
#88131=CARTESIAN_POINT('',(16.0572936004958,4.61234089134698,-5.20507760384135));
#88132=CARTESIAN_POINT('',(14.0010657378079,9.11485186254263,-5.20507760384135));
#88133=CARTESIAN_POINT('Origin',(-1.05198826215219,-0.480426941701518,-9.70476622208446));
#88134=CARTESIAN_POINT('',(14.1656160094783,3.73398019712069,2.87709523867187));
#88135=CARTESIAN_POINT('Ctrl Pts',(16.0572936004958,4.61234089134702,-5.20507760384136));
#88136=CARTESIAN_POINT('Ctrl Pts',(15.7183902268811,4.45528963367599,-3.75496347264913));
#88137=CARTESIAN_POINT('Ctrl Pts',(15.3792722311841,4.29799199952221,-2.30492612391988));
#88138=CARTESIAN_POINT('Ctrl Pts',(15.039883904257,4.14038936594967,-0.854985236809349));
#88139=CARTESIAN_POINT('Ctrl Pts',(14.7486760715879,4.00516043288306,0.38911808005159));
#88140=CARTESIAN_POINT('Ctrl Pts',(14.4572691812803,3.86970690561884,1.63315045290804));
#88141=CARTESIAN_POINT('Ctrl Pts',(14.1656160094783,3.73398019712069,2.87709523867187));
#88142=CARTESIAN_POINT('',(12.0984596413753,8.26042125720544,2.87709523867187));
#88143=CARTESIAN_POINT('Origin',(-0.92225862834957,-0.42118140307714,-1.05545232631937));
#88144=CARTESIAN_POINT('Ctrl Pts',(12.0984596413753,8.26042125720544,2.87709523867187));
#88145=CARTESIAN_POINT('Ctrl Pts',(12.4864428546168,8.43425938238591,1.23307977231272));
#88146=CARTESIAN_POINT('Ctrl Pts',(12.8737856194689,8.60808505767906,-0.411088229465946));
#88147=CARTESIAN_POINT('Ctrl Pts',(13.2606377386196,8.7819066131822,-2.05537200357358));
#88148=CARTESIAN_POINT('Ctrl Pts',(13.5076384645677,8.89288972085904,-3.1052286949651));
#88149=CARTESIAN_POINT('Ctrl Pts',(13.7544379950536,9.00387103738414,-4.15513295741834));
#88150=CARTESIAN_POINT('Ctrl Pts',(14.0010657378079,9.11485186254263,-5.20507760384135));
#88151=CARTESIAN_POINT('',(-14.0010657378077,9.11485186254283,-5.20507760384135));
#88152=CARTESIAN_POINT('',(-16.0572936004957,4.61234089134721,-5.20507760384135));
#88153=CARTESIAN_POINT('Origin',(1.05198826173568,-0.480426941512203,-9.7047662219679));
#88154=CARTESIAN_POINT('',(-12.0984596413752,8.26042125720561,2.87709523867187));
#88155=CARTESIAN_POINT('Ctrl Pts',(-14.0010657378077,9.11485186254283,-5.20507760384135));
#88156=CARTESIAN_POINT('Ctrl Pts',(-13.5855255950981,8.92786159368845,-3.43603838975674));
#88157=CARTESIAN_POINT('Ctrl Pts',(-13.1695007029774,8.74087017903734,-1.66711304381579));
#88158=CARTESIAN_POINT('Ctrl Pts',(-12.7528393518526,8.55387043894279,0.101661445498907));
#88159=CARTESIAN_POINT('Ctrl Pts',(-12.534897354391,8.45605695859243,1.02684983702997));
#88160=CARTESIAN_POINT('Ctrl Pts',(-12.316780375612,8.35824112629394,1.95199680280524));
#88161=CARTESIAN_POINT('Ctrl Pts',(-12.0984596413752,8.26042125720561,2.87709523867187));
#88162=CARTESIAN_POINT('',(-14.1656160094783,3.73398019712089,2.87709523867187));
#88163=CARTESIAN_POINT('Origin',(0.922258628312644,-0.421181403062295,-1.05545232630926));
#88164=CARTESIAN_POINT('Ctrl Pts',(-14.1656160094783,3.73398019712093,2.87709523867186));
#88165=CARTESIAN_POINT('Ctrl Pts',(-14.5510690703717,3.91335858314142,1.23307977231272));
#88166=CARTESIAN_POINT('Ctrl Pts',(-14.9360933177658,4.09226110350664,-0.411088229465959));
#88167=CARTESIAN_POINT('Ctrl Pts',(-15.3207931456275,4.27079551583136,-2.05537199759547));
#88168=CARTESIAN_POINT('Ctrl Pts',(-15.5664196600929,4.38478773063213,-3.1052286949651));
#88169=CARTESIAN_POINT('Ctrl Pts',(-15.8119130644899,4.49862906435458,-4.15513295741812));
#88170=CARTESIAN_POINT('Ctrl Pts',(-16.0572936004957,4.61234089134724,-5.20507760384135));
#88171=CARTESIAN_POINT('',(2.47490798157382,16.5222636691604,-5.20507760384135));
#88172=CARTESIAN_POINT('',(-2.47490798157382,16.5222636691604,-5.20507760384135));
#88173=CARTESIAN_POINT('Origin',(-1.52378110129803E-13,-1.15649874592685,
-9.70476622200868));
#88174=CARTESIAN_POINT('',(2.48806170143598,14.4366489882634,2.87709523867187));
#88175=CARTESIAN_POINT('Ctrl Pts',(2.47490798157379,16.5222636691604,-5.20507760384135));
#88176=CARTESIAN_POINT('Ctrl Pts',(2.47698128110552,16.1487448669395,-3.75496347264913));
#88177=CARTESIAN_POINT('Ctrl Pts',(2.47918953533373,15.7749284891158,-2.30492612391988));
#88178=CARTESIAN_POINT('Ctrl Pts',(2.48156292714035,15.4007395080185,-0.854985236809348));
#88179=CARTESIAN_POINT('Ctrl Pts',(2.4835993857609,15.0796714171367,0.389118080051589));
#88180=CARTESIAN_POINT('Ctrl Pts',(2.48575745091808,14.7583289572565,1.63315045290804));
#88181=CARTESIAN_POINT('Ctrl Pts',(2.48806170143596,14.4366489882634,2.87709523867187));
#88182=CARTESIAN_POINT('',(-2.48806170143598,14.4366489882634,2.87709523867187));
#88183=CARTESIAN_POINT('Origin',(-1.14630527292547E-13,-1.01388103426158,
-1.05545232629072));
#88184=CARTESIAN_POINT('Ctrl Pts',(-2.48806170143596,14.4366489882634,2.87709523867187));
#88185=CARTESIAN_POINT('Ctrl Pts',(-2.48501637053932,14.8617858997204,1.23307977231273));
#88186=CARTESIAN_POINT('Ctrl Pts',(-2.48222576670286,15.2863350669608,-0.411088229465946));
#88187=CARTESIAN_POINT('Ctrl Pts',(-2.47963523697349,15.7104362142084,-2.05537199759546));
#88188=CARTESIAN_POINT('Ctrl Pts',(-2.47798121286961,15.9812200280671,-3.10522869496509));
#88189=CARTESIAN_POINT('Ctrl Pts',(-2.47640913910131,16.2518200824836,-4.15513295741812));
#88190=CARTESIAN_POINT('Ctrl Pts',(-2.47490798157379,16.5222636691604,-5.20507760384135));
#88191=CARTESIAN_POINT('',(11.0146352192429,12.5613764077639,-5.20507760384135));
#88192=CARTESIAN_POINT('',(6.85058505338072,15.2374489563349,-5.20507760384135));
#88193=CARTESIAN_POINT('Origin',(-0.625250427241271,-0.972908655507905,
-9.7047662219421));
#88194=CARTESIAN_POINT('',(9.89813240656923,10.7997342514759,2.87709523867187));
#88195=CARTESIAN_POINT('Ctrl Pts',(11.0146352192428,12.5613764077639,-5.20507760384136));
#88196=CARTESIAN_POINT('Ctrl Pts',(10.7749172616532,12.1837760065475,-3.46868155296237));
#88197=CARTESIAN_POINT('Ctrl Pts',(10.5351317085667,11.8057133276335,-1.73239525071041));
#88198=CARTESIAN_POINT('Ctrl Pts',(10.2952515367979,11.427047819608,0.00374645021393172));
#88199=CARTESIAN_POINT('Ctrl Pts',(10.1629096012127,11.2181379880787,0.961576151002431));
#88200=CARTESIAN_POINT('Ctrl Pts',(10.0305386804728,11.0090438751527,1.91936169771154));
#88201=CARTESIAN_POINT('Ctrl Pts',(9.89813240656922,10.7997342514759,2.87709523867187));
#88202=CARTESIAN_POINT('',(5.71195101409927,13.4900296757646,2.87709523867187));
#88203=CARTESIAN_POINT('Origin',(-0.548145471286394,-0.852931002129471,
-1.05545232634732));
#88204=CARTESIAN_POINT('Ctrl Pts',(5.71195101409927,13.4900296757646,2.87709523867187));
#88205=CARTESIAN_POINT('Ctrl Pts',(5.94435927681535,13.8460311742793,1.23307977231273));
#88206=CARTESIAN_POINT('Ctrl Pts',(6.17623549097855,14.2016759467416,-0.411088229465952));
#88207=CARTESIAN_POINT('Ctrl Pts',(6.40770117419705,14.5570519890308,-2.05537199759546));
#88208=CARTESIAN_POINT('Ctrl Pts',(6.55548941029612,14.7839555961293,-3.10522869496509));
#88209=CARTESIAN_POINT('Ctrl Pts',(6.70310935753085,15.0107489206444,-4.15513295741812));
#88210=CARTESIAN_POINT('Ctrl Pts',(6.85058505338072,15.2374489563349,-5.20507760384135));
#88211=CARTESIAN_POINT('',(-6.8505850533805,15.237448956335,-5.20507760384135));
#88212=CARTESIAN_POINT('',(-11.0146352192427,12.5613764077641,-5.20507760384135));
#88213=CARTESIAN_POINT('Origin',(0.625250427357654,-0.972908655687406,-9.70476622199673));
#88214=CARTESIAN_POINT('',(-5.71195101409907,13.4900296757646,2.87709523867187));
#88215=CARTESIAN_POINT('Ctrl Pts',(-6.85058505338051,15.237448956335,-5.20507760384135));
#88216=CARTESIAN_POINT('Ctrl Pts',(-6.6469013722571,14.9243458547414,-3.75496347264912));
#88217=CARTESIAN_POINT('Ctrl Pts',(-6.44294327850138,14.6110653786382,-2.30492612391988));
#88218=CARTESIAN_POINT('Ctrl Pts',(-6.23864481763592,14.2975607288301,-0.854985236809342));
#88219=CARTESIAN_POINT('Ctrl Pts',(-6.0633491245137,14.0285620557497,0.389118080051595));
#88220=CARTESIAN_POINT('Ctrl Pts',(-5.88780279438331,13.7593983142375,1.63315045290805));
#88221=CARTESIAN_POINT('Ctrl Pts',(-5.71195101409905,13.4900296757646,2.87709523867188));
#88222=CARTESIAN_POINT('',(-9.89813240656907,10.7997342514761,2.87709523867187));
#88223=CARTESIAN_POINT('Origin',(0.548145471174728,-0.85293100195315,-1.0554523262942));
#88224=CARTESIAN_POINT('Ctrl Pts',(-9.89813240656907,10.7997342514761,2.87709523867187));
#88225=CARTESIAN_POINT('Ctrl Pts',(-10.1254168785343,11.1590286103616,1.23307977231272));
#88226=CARTESIAN_POINT('Ctrl Pts',(-10.3525978820251,11.5176908115025,-0.411088229465944));
#88227=CARTESIAN_POINT('Ctrl Pts',(-10.5797049814101,11.8758679471799,-2.05537200295315));
#88228=CARTESIAN_POINT('Ctrl Pts',(-10.7247103095276,12.1045600189986,-3.1052286949651));
#88229=CARTESIAN_POINT('Ctrl Pts',(-10.8696852315395,12.333053198008,-4.15513295741812));
#88230=CARTESIAN_POINT('Ctrl Pts',(-11.0146352192427,12.5613764077641,-5.20507760384135));
#88231=CARTESIAN_POINT('Origin',(0.,15.3635472745355,-5.5));
#88232=CARTESIAN_POINT('Origin',(0.,13.3046975771901,2.58898520239593));
#88233=CARTESIAN_POINT('Origin',(0.,15.3635472745355,-5.5));
#88234=CARTESIAN_POINT('Origin',(0.,15.3635472745355,-5.5));
#88235=CARTESIAN_POINT('Origin',(0.,15.3635472745355,-5.5));
#88236=CARTESIAN_POINT('Origin',(0.,13.3046975771901,2.58898520239593));
#88237=CARTESIAN_POINT('Origin',(0.,15.3635472745355,-5.5));
#88238=CARTESIAN_POINT('Origin',(0.,13.3046975771901,2.58898520239593));
#88239=CARTESIAN_POINT('Origin',(8.30616075752262,12.9246384215219,-5.5));
#88240=CARTESIAN_POINT('Origin',(7.1930625741316,11.1926238400616,2.58898520239593));
#88241=CARTESIAN_POINT('Origin',(8.30616075752262,12.9246384215219,-5.5));
#88242=CARTESIAN_POINT('Origin',(8.30616075752262,12.9246384215219,-5.5));
#88243=CARTESIAN_POINT('Origin',(8.30616075752262,12.9246384215219,-5.5));
#88244=CARTESIAN_POINT('Origin',(7.1930625741316,11.1926238400616,2.58898520239593));
#88245=CARTESIAN_POINT('Origin',(8.30616075752262,12.9246384215219,-5.5));
#88246=CARTESIAN_POINT('Origin',(7.1930625741316,11.1926238400616,2.58898520239593));
#88247=CARTESIAN_POINT('Origin',(-13.9751741630591,6.38224819080644,-5.5));
#88248=CARTESIAN_POINT('Origin',(-12.1023786047278,5.52697111701475,2.58898520239593));
#88249=CARTESIAN_POINT('Origin',(-13.9751741630591,6.38224819080644,-5.5));
#88250=CARTESIAN_POINT('Origin',(-13.9751741630591,6.38224819080644,-5.5));
#88251=CARTESIAN_POINT('Origin',(-13.9751741630591,6.38224819080644,-5.5));
#88252=CARTESIAN_POINT('Origin',(-12.1023786047278,5.52697111701475,2.58898520239593));
#88253=CARTESIAN_POINT('Origin',(-13.9751741630591,6.38224819080644,-5.5));
#88254=CARTESIAN_POINT('Origin',(-12.1023786047278,5.52697111701475,2.58898520239593));
#88255=CARTESIAN_POINT('Origin',(-8.30616075752243,12.924638421522,-5.5));
#88256=CARTESIAN_POINT('Origin',(-7.19306257413143,11.1926238400618,2.58898520239593));
#88257=CARTESIAN_POINT('Origin',(-8.30616075752243,12.924638421522,-5.5));
#88258=CARTESIAN_POINT('Origin',(-8.30616075752243,12.924638421522,-5.5));
#88259=CARTESIAN_POINT('Origin',(-8.30616075752243,12.924638421522,-5.5));
#88260=CARTESIAN_POINT('Origin',(-7.19306257413143,11.1926238400618,2.58898520239593));
#88261=CARTESIAN_POINT('Origin',(-8.30616075752243,12.924638421522,-5.5));
#88262=CARTESIAN_POINT('Origin',(-7.19306257413143,11.1926238400618,2.58898520239593));
#88263=CARTESIAN_POINT('Origin',(-15.2071685156867,-2.18646074567933,-5.5));
#88264=CARTESIAN_POINT('Origin',(-13.1692749396441,-1.89345588397264,2.58898520239593));
#88265=CARTESIAN_POINT('Origin',(-15.2071685156867,-2.18646074567933,-5.5));
#88266=CARTESIAN_POINT('Origin',(-15.2071685156867,-2.18646074567933,-5.5));
#88267=CARTESIAN_POINT('Origin',(-15.2071685156867,-2.18646074567933,-5.5));
#88268=CARTESIAN_POINT('Origin',(-13.1692749396441,-1.89345588397264,2.58898520239593));
#88269=CARTESIAN_POINT('Origin',(-15.2071685156867,-2.18646074567933,-5.5));
#88270=CARTESIAN_POINT('Origin',(-13.1692749396441,-1.89345588397264,2.58898520239593));
#88271=CARTESIAN_POINT('Origin',(-11.6109943133018,-10.0609838442053,-5.5));
#88272=CARTESIAN_POINT('Origin',(-10.0550195308737,-8.71272402031869,2.58898520239593));
#88273=CARTESIAN_POINT('Origin',(-11.6109943133018,-10.0609838442053,-5.5));
#88274=CARTESIAN_POINT('Origin',(-11.6109943133018,-10.0609838442053,-5.5));
#88275=CARTESIAN_POINT('Origin',(-11.6109943133018,-10.0609838442053,-5.5));
#88276=CARTESIAN_POINT('Origin',(-10.0550195308737,-8.71272402031869,2.58898520239593));
#88277=CARTESIAN_POINT('Origin',(-11.6109943133018,-10.0609838442053,-5.5));
#88278=CARTESIAN_POINT('Origin',(-10.0550195308737,-8.71272402031869,2.58898520239593));
#88279=CARTESIAN_POINT('Origin',(-4.32841145580919,-14.741215659711,-5.5));
#88280=CARTESIAN_POINT('Origin',(-3.74836646642385,-12.7657638413797,2.58898520239593));
#88281=CARTESIAN_POINT('Origin',(-4.32841145580919,-14.741215659711,-5.5));
#88282=CARTESIAN_POINT('Origin',(-4.32841145580919,-14.741215659711,-5.5));
#88283=CARTESIAN_POINT('Origin',(-4.32841145580919,-14.741215659711,-5.5));
#88284=CARTESIAN_POINT('Origin',(-3.74836646642385,-12.7657638413797,2.58898520239593));
#88285=CARTESIAN_POINT('Origin',(-4.32841145580919,-14.741215659711,-5.5));
#88286=CARTESIAN_POINT('Origin',(-3.74836646642385,-12.7657638413797,2.58898520239593));
#88287=CARTESIAN_POINT('Origin',(4.32841145580897,-14.741215659711,-5.5));
#88288=CARTESIAN_POINT('Origin',(3.74836646642367,-12.7657638413798,2.58898520239593));
#88289=CARTESIAN_POINT('Origin',(4.32841145580897,-14.741215659711,-5.5));
#88290=CARTESIAN_POINT('Origin',(4.32841145580897,-14.741215659711,-5.5));
#88291=CARTESIAN_POINT('Origin',(4.32841145580897,-14.741215659711,-5.5));
#88292=CARTESIAN_POINT('Origin',(3.74836646642367,-12.7657638413798,2.58898520239593));
#88293=CARTESIAN_POINT('Origin',(4.32841145580897,-14.741215659711,-5.5));
#88294=CARTESIAN_POINT('Origin',(3.74836646642367,-12.7657638413798,2.58898520239593));
#88295=CARTESIAN_POINT('Origin',(11.6109943133017,-10.0609838442055,-5.5));
#88296=CARTESIAN_POINT('Origin',(10.0550195308735,-8.71272402031884,2.58898520239593));
#88297=CARTESIAN_POINT('Origin',(11.6109943133017,-10.0609838442055,-5.5));
#88298=CARTESIAN_POINT('Origin',(11.6109943133017,-10.0609838442055,-5.5));
#88299=CARTESIAN_POINT('Origin',(11.6109943133017,-10.0609838442055,-5.5));
#88300=CARTESIAN_POINT('Origin',(10.0550195308735,-8.71272402031884,2.58898520239593));
#88301=CARTESIAN_POINT('Origin',(11.6109943133017,-10.0609838442055,-5.5));
#88302=CARTESIAN_POINT('Origin',(10.0550195308735,-8.71272402031884,2.58898520239593));
#88303=CARTESIAN_POINT('Origin',(15.2071685156866,-2.18646074567955,-5.5));
#88304=CARTESIAN_POINT('Origin',(13.1692749396441,-1.89345588397283,2.58898520239593));
#88305=CARTESIAN_POINT('Origin',(15.2071685156866,-2.18646074567955,-5.5));
#88306=CARTESIAN_POINT('Origin',(15.2071685156866,-2.18646074567955,-5.5));
#88307=CARTESIAN_POINT('Origin',(15.2071685156866,-2.18646074567955,-5.5));
#88308=CARTESIAN_POINT('Origin',(13.1692749396441,-1.89345588397283,2.58898520239593));
#88309=CARTESIAN_POINT('Origin',(15.2071685156866,-2.18646074567955,-5.5));
#88310=CARTESIAN_POINT('Origin',(13.1692749396441,-1.89345588397283,2.58898520239593));
#88311=CARTESIAN_POINT('Origin',(13.9751741630592,6.38224819080624,-5.5));
#88312=CARTESIAN_POINT('Origin',(12.1023786047279,5.52697111701458,2.58898520239593));
#88313=CARTESIAN_POINT('Origin',(13.9751741630592,6.38224819080624,-5.5));
#88314=CARTESIAN_POINT('Origin',(13.9751741630592,6.38224819080624,-5.5));
#88315=CARTESIAN_POINT('Origin',(13.9751741630592,6.38224819080624,-5.5));
#88316=CARTESIAN_POINT('Origin',(12.1023786047279,5.52697111701458,2.58898520239593));
#88317=CARTESIAN_POINT('Origin',(13.9751741630592,6.38224819080624,-5.5));
#88318=CARTESIAN_POINT('Origin',(12.1023786047279,5.52697111701458,2.58898520239593));
#88319=CARTESIAN_POINT('Origin',(0.,0.,3.975));
#88320=CARTESIAN_POINT('',(8.775,-1.0746275662518E-15,4.25));
#88321=CARTESIAN_POINT('Origin',(0.,0.,4.25));
#88322=CARTESIAN_POINT('',(8.5,-1.04094977927525E-15,3.975));
#88323=CARTESIAN_POINT('Origin',(8.775,-1.0746275662518E-15,3.975));
#88324=CARTESIAN_POINT('',(-8.5,1.04094977927525E-15,3.975));
#88325=CARTESIAN_POINT('Origin',(0.,0.,3.975));
#88326=CARTESIAN_POINT('Origin',(0.,0.,3.975));
#88327=CARTESIAN_POINT('Origin',(0.,0.,-7.475));
#88328=CARTESIAN_POINT('',(-8.775,-1.0746275662518E-15,-7.75));
#88329=CARTESIAN_POINT('Origin',(0.,0.,-7.75));
#88330=CARTESIAN_POINT('',(-8.5,-1.04094977927525E-15,-7.475));
#88331=CARTESIAN_POINT('Origin',(-8.775,-1.0746275662518E-15,-7.475));
#88332=CARTESIAN_POINT('Origin',(0.,0.,-7.475));
#88333=CARTESIAN_POINT('Origin',(0.,0.,1.91101479760404));
#88334=CARTESIAN_POINT('',(-11.9728634517814,-1.46625289028525E-15,2.24999999999999));
#88335=CARTESIAN_POINT('Origin',(0.,0.,2.24999999999999));
#88336=CARTESIAN_POINT('',(-10.6410293263727,-1.30315025041754E-15,1.91101479760404));
#88337=CARTESIAN_POINT('',(-10.6410293263727,-1.30315025041754E-15,1.91101479760404));
#88338=CARTESIAN_POINT('',(10.6410293263727,1.42921843500653E-15,1.91101479760404));
#88339=CARTESIAN_POINT('Origin',(0.,0.,1.91101479760404));
#88340=CARTESIAN_POINT('Origin',(0.,0.,1.91101479760404));
#88341=CARTESIAN_POINT('Origin',(0.,0.,-6.17797040479189));
#88342=CARTESIAN_POINT('',(-12.6998790237181,1.63683793952935E-15,-6.17797040479189));
#88343=CARTESIAN_POINT('',(12.6998790237181,-1.5552866195955E-15,-6.17797040479189));
#88344=CARTESIAN_POINT('Origin',(0.,0.,-6.17797040479189));
#88345=CARTESIAN_POINT('',(12.6998790237181,-1.5552866195955E-15,-6.17797040479189));
#88346=CARTESIAN_POINT('Origin',(0.,0.,-6.17797040479189));
#88347=CARTESIAN_POINT('Origin',(0.,0.,-5.83898520239594));
#88348=CARTESIAN_POINT('',(-14.0317131491268,-1.7183892594632E-15,-5.83898520239594));
#88349=CARTESIAN_POINT('',(-14.0317131491268,-1.7183892594632E-15,-5.83898520239594));
#88350=CARTESIAN_POINT('Origin',(0.,0.,-5.83898520239594));
#88351=CARTESIAN_POINT('Origin',(0.,0.,4.25));
#88352=CARTESIAN_POINT('',(-14.0317131491268,-1.7183892594632E-15,-7.75));
#88353=CARTESIAN_POINT('',(-14.0317131491268,-1.7183892594632E-15,4.25));
#88354=CARTESIAN_POINT('Origin',(0.,0.,-7.75));
#88355=CARTESIAN_POINT('Origin',(0.,0.,4.25));
#88356=CARTESIAN_POINT('',(-8.5,-1.04094977927525E-15,4.25));
#88357=CARTESIAN_POINT('Origin',(0.,0.,4.25));
#88358=CARTESIAN_POINT('',(-11.9728634517814,-1.46625289028525E-15,4.25));
#88359=CARTESIAN_POINT('Origin',(0.,0.,4.25));
#88360=CARTESIAN_POINT('',(-11.9728634517814,-1.46625289028524E-15,4.25));
#88361=CARTESIAN_POINT('Origin',(0.,11.9728634517814,4.25));
#88362=CARTESIAN_POINT('Origin',(0.,8.5,-7.75));
#88363=CARTESIAN_POINT('Origin',(0.,15.3635472745355,-5.5));
#88364=CARTESIAN_POINT('',(-3.21052746786287E-16,15.8452898878137,3.2356296922704));
#88365=CARTESIAN_POINT('Origin',(0.,13.3046975771901,2.58898520239593));
#88366=CARTESIAN_POINT('',(-3.21052746786287E-16,17.9041395851591,-4.85335551012554));
#88367=CARTESIAN_POINT('',(-3.21052746786287E-16,17.9041395851591,-4.85335551012554));
#88368=CARTESIAN_POINT('Origin',(0.,15.3635472745355,-5.5));
#88369=CARTESIAN_POINT('Origin',(0.,15.3635472745355,-5.5));
#88370=CARTESIAN_POINT('Origin',(0.,13.3046975771901,2.58898520239593));
#88371=CARTESIAN_POINT('Origin',(8.30616075752262,12.9246384215219,-5.5));
#88372=CARTESIAN_POINT('',(8.56661047776854,13.3299060968575,3.2356296922704));
#88373=CARTESIAN_POINT('Origin',(7.1930625741316,11.1926238400616,2.58898520239593));
#88374=CARTESIAN_POINT('',(9.67970866115956,15.0619206783177,-4.85335551012554));
#88375=CARTESIAN_POINT('',(9.67970866115956,15.0619206783177,-4.85335551012554));
#88376=CARTESIAN_POINT('Origin',(8.30616075752262,12.9246384215219,-5.5));
#88377=CARTESIAN_POINT('Origin',(8.30616075752262,12.9246384215219,-5.5));
#88378=CARTESIAN_POINT('Origin',(7.1930625741316,11.1926238400616,2.58898520239593));
#88379=CARTESIAN_POINT('Origin',(13.9751741630592,6.38224819080624,-5.5));
#88380=CARTESIAN_POINT('',(14.4133826576228,6.58237130476475,3.2356296922704));
#88381=CARTESIAN_POINT('Origin',(12.1023786047279,5.52697111701458,2.58898520239593));
#88382=CARTESIAN_POINT('',(16.2861782159541,7.43764837855642,-4.85335551012554));
#88383=CARTESIAN_POINT('',(16.2861782159541,7.43764837855642,-4.85335551012554));
#88384=CARTESIAN_POINT('Origin',(13.9751741630592,6.38224819080624,-5.5));
#88385=CARTESIAN_POINT('Origin',(13.9751741630592,6.38224819080624,-5.5));
#88386=CARTESIAN_POINT('Origin',(12.1023786047279,5.52697111701458,2.58898520239593));
#88387=CARTESIAN_POINT('Origin',(15.2071685156866,-2.18646074567955,-5.5));
#88388=CARTESIAN_POINT('',(15.6840076837771,-2.25501986777759,3.2356296922704));
#88389=CARTESIAN_POINT('Origin',(13.1692749396441,-1.89345588397283,2.58898520239593));
#88390=CARTESIAN_POINT('',(17.7219012598197,-2.54802472948431,-4.85335551012554));
#88391=CARTESIAN_POINT('',(17.7219012598196,-2.5480247294843,-4.85335551012554));
#88392=CARTESIAN_POINT('Origin',(15.2071685156866,-2.18646074567955,-5.5));
#88393=CARTESIAN_POINT('Origin',(15.2071685156866,-2.18646074567955,-5.5));
#88394=CARTESIAN_POINT('Origin',(13.1692749396441,-1.89345588397283,2.58898520239593));
#88395=CARTESIAN_POINT('Origin',(11.6109943133017,-10.0609838442055,-5.5));
#88396=CARTESIAN_POINT('',(11.975071088235,-10.3764581655096,3.2356296922704));
#88397=CARTESIAN_POINT('Origin',(10.0550195308735,-8.71272402031884,2.58898520239593));
#88398=CARTESIAN_POINT('',(13.5310458706632,-11.7247179893962,-4.85335551012554));
#88399=CARTESIAN_POINT('',(13.5310458706632,-11.7247179893962,-4.85335551012554));
#88400=CARTESIAN_POINT('Origin',(11.6109943133017,-10.0609838442055,-5.5));
#88401=CARTESIAN_POINT('Origin',(11.6109943133017,-10.0609838442055,-5.5));
#88402=CARTESIAN_POINT('Origin',(10.0550195308735,-8.71272402031884,2.58898520239593));
#88403=CARTESIAN_POINT('Origin',(4.32841145580897,-14.741215659711,-5.5));
#88404=CARTESIAN_POINT('',(4.46413403398731,-15.2034443122421,3.2356296922704));
#88405=CARTESIAN_POINT('Origin',(3.74836646642367,-12.7657638413798,2.58898520239593));
#88406=CARTESIAN_POINT('',(5.04417902337261,-17.1788961305734,-4.85335551012554));
#88407=CARTESIAN_POINT('',(5.04417902337261,-17.1788961305733,-4.85335551012554));
#88408=CARTESIAN_POINT('Origin',(4.32841145580897,-14.741215659711,-5.5));
#88409=CARTESIAN_POINT('Origin',(4.32841145580897,-14.741215659711,-5.5));
#88410=CARTESIAN_POINT('Origin',(3.74836646642367,-12.7657638413798,2.58898520239593));
#88411=CARTESIAN_POINT('Origin',(-4.32841145580919,-14.741215659711,-5.5));
#88412=CARTESIAN_POINT('',(-4.46413403398752,-15.2034443122421,3.2356296922704));
#88413=CARTESIAN_POINT('Origin',(-3.74836646642385,-12.7657638413797,2.58898520239593));
#88414=CARTESIAN_POINT('',(-5.04417902337286,-17.1788961305733,-4.85335551012554));
#88415=CARTESIAN_POINT('',(-5.04417902337286,-17.1788961305733,-4.85335551012554));
#88416=CARTESIAN_POINT('Origin',(-4.32841145580919,-14.741215659711,-5.5));
#88417=CARTESIAN_POINT('Origin',(-4.32841145580919,-14.741215659711,-5.5));
#88418=CARTESIAN_POINT('Origin',(-3.74836646642385,-12.7657638413797,2.58898520239593));
#88419=CARTESIAN_POINT('Origin',(-11.6109943133018,-10.0609838442053,-5.5));
#88420=CARTESIAN_POINT('',(-11.9750710882351,-10.3764581655094,3.2356296922704));
#88421=CARTESIAN_POINT('Origin',(-10.0550195308737,-8.71272402031869,2.58898520239593));
#88422=CARTESIAN_POINT('',(-13.5310458706633,-11.724717989396,-4.85335551012554));
#88423=CARTESIAN_POINT('',(-13.5310458706633,-11.724717989396,-4.85335551012554));
#88424=CARTESIAN_POINT('Origin',(-11.6109943133018,-10.0609838442053,-5.5));
#88425=CARTESIAN_POINT('Origin',(-11.6109943133018,-10.0609838442053,-5.5));
#88426=CARTESIAN_POINT('Origin',(-10.0550195308737,-8.71272402031869,2.58898520239593));
#88427=CARTESIAN_POINT('Origin',(-15.2071685156867,-2.18646074567933,-5.5));
#88428=CARTESIAN_POINT('',(-15.6840076837772,-2.25501986777736,3.2356296922704));
#88429=CARTESIAN_POINT('Origin',(-13.1692749396441,-1.89345588397264,2.58898520239593));
#88430=CARTESIAN_POINT('',(-17.7219012598197,-2.54802472948405,-4.85335551012554));
#88431=CARTESIAN_POINT('',(-17.7219012598197,-2.54802472948405,-4.85335551012554));
#88432=CARTESIAN_POINT('Origin',(-15.2071685156867,-2.18646074567933,-5.5));
#88433=CARTESIAN_POINT('Origin',(-15.2071685156867,-2.18646074567933,-5.5));
#88434=CARTESIAN_POINT('Origin',(-13.1692749396441,-1.89345588397264,2.58898520239593));
#88435=CARTESIAN_POINT('Origin',(-13.9751741630591,6.38224819080644,-5.5));
#88436=CARTESIAN_POINT('',(-14.4133826576227,6.58237130476496,3.2356296922704));
#88437=CARTESIAN_POINT('Origin',(-12.1023786047278,5.52697111701475,2.58898520239593));
#88438=CARTESIAN_POINT('',(-16.286178215954,7.43764837855665,-4.85335551012554));
#88439=CARTESIAN_POINT('',(-16.286178215954,7.43764837855665,-4.85335551012554));
#88440=CARTESIAN_POINT('Origin',(-13.9751741630591,6.38224819080644,-5.5));
#88441=CARTESIAN_POINT('Origin',(-13.9751741630591,6.38224819080644,-5.5));
#88442=CARTESIAN_POINT('Origin',(-12.1023786047278,5.52697111701475,2.58898520239593));
#88443=CARTESIAN_POINT('Origin',(-8.30616075752243,12.924638421522,-5.5));
#88444=CARTESIAN_POINT('',(-8.56661047776834,13.3299060968576,3.2356296922704));
#88445=CARTESIAN_POINT('Origin',(-7.19306257413143,11.1926238400618,2.58898520239593));
#88446=CARTESIAN_POINT('',(-9.67970866115934,15.0619206783178,-4.85335551012554));
#88447=CARTESIAN_POINT('',(-9.67970866115934,15.0619206783178,-4.85335551012554));
#88448=CARTESIAN_POINT('Origin',(-8.30616075752243,12.924638421522,-5.5));
#88449=CARTESIAN_POINT('Origin',(-8.30616075752243,12.924638421522,-5.5));
#88450=CARTESIAN_POINT('Origin',(-7.19306257413143,11.1926238400618,2.58898520239593));
#88471=UNCERTAINTY_MEASURE_WITH_UNIT(LENGTH_MEASURE(0.01),#88484,
'DISTANCE_ACCURACY_VALUE',
'Maximum model space distance between geometric entities at asserted c
onnectivities');
#88472=UNCERTAINTY_MEASURE_WITH_UNIT(LENGTH_MEASURE(0.01),#88484,
'DISTANCE_ACCURACY_VALUE',
'Maximum model space distance between geometric entities at asserted c
onnectivities');
#88482=(
GEOMETRIC_REPRESENTATION_CONTEXT(3)
GLOBAL_UNCERTAINTY_ASSIGNED_CONTEXT((#88471))
GLOBAL_UNIT_ASSIGNED_CONTEXT((#88484,#88486,#88487))
REPRESENTATION_CONTEXT('','3D')
);
#88483=(
GEOMETRIC_REPRESENTATION_CONTEXT(3)
GLOBAL_UNCERTAINTY_ASSIGNED_CONTEXT((#88472))
GLOBAL_UNIT_ASSIGNED_CONTEXT((#88484,#88486,#88487))
REPRESENTATION_CONTEXT('','3D')
);
#88484=(
LENGTH_UNIT()
NAMED_UNIT(*)
SI_UNIT(.MILLI.,.METRE.)
);
#88486=(
NAMED_UNIT(*)
PLANE_ANGLE_UNIT()
SI_UNIT($,.RADIAN.)
);
#88487=(
NAMED_UNIT(*)
SI_UNIT($,.STERADIAN.)
SOLID_ANGLE_UNIT()
);
#88497=SHAPE_DEFINITION_REPRESENTATION(#88507,#88528);
#88507=PRODUCT_DEFINITION_SHAPE('',$,#88539);
#88528=SHAPE_REPRESENTATION('',(#14115),#88482);
#88529=PRODUCT_DEFINITION_CONTEXT('part definition',#88561,'design');
#88539=PRODUCT_DEFINITION('Tapered-Roller Bearing with Steel Ring',
'Tapered-Roller Bearing with Steel Ring',#88549,#88529);
#88549=PRODUCT_DEFINITION_FORMATION('',$,#88572);
#88561=APPLICATION_CONTEXT(
'Core Data for Automotive Mechanical Design Process');
#88562=PRODUCT_CONTEXT('part definition',#88561,'mechanical');
#88572=PRODUCT('Tapered-Roller Bearing with Steel Ring',
'Tapered-Roller Bearing with Steel Ring',$,(#88562));
#88574=PRESENTATION_STYLE_ASSIGNMENT((#88576));
#88576=SURFACE_STYLE_USAGE(.BOTH.,#88578);
#88578=SURFACE_SIDE_STYLE('',(#88580));
#88580=SURFACE_STYLE_FILL_AREA(#88582);
#88582=FILL_AREA_STYLE('Opaque(160,160,160)',(#88584));
#88584=FILL_AREA_STYLE_COLOUR('Opaque(160,160,160)',#88586);
#88586=COLOUR_RGB('Opaque(160,160,160)', 0.66274510, 0.83137255, 0.94901961);
ENDSEC;
END-ISO-10303-21;
